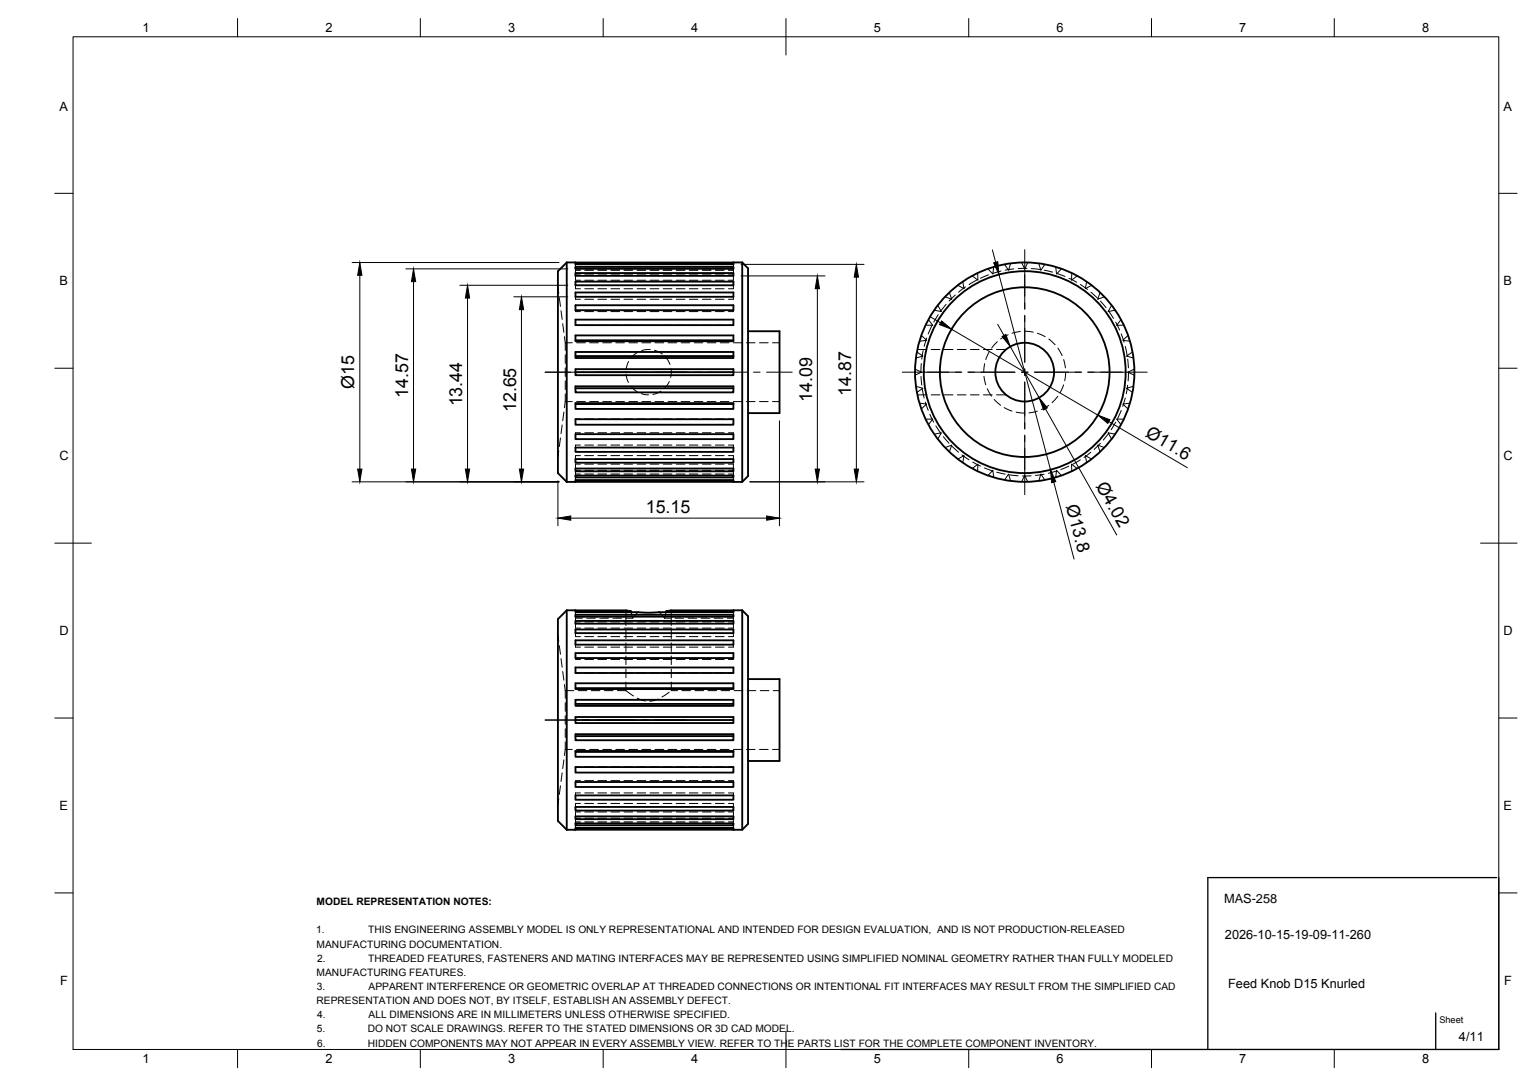
ISO-10303-21;
HEADER;
/* Generated by software containing ST-Developer
 * from STEP Tools, Inc. (www.steptools.com) 
 */

FILE_DESCRIPTION(
/* description */ (''),
/* implementation_level */ '2;1');

FILE_NAME(
/* name */ 'Feed Knob D15 Knurled.step',
/* time_stamp */ '2026-10-15T12:29:06-07:00',
/* author */ (''),
/* organization */ (''),
/* preprocessor_version */ 'ST-DEVELOPER v20.2',
/* originating_system */ 'Autodesk Translation Framework v15.15.0.0',
/* authorisation */ '');

FILE_SCHEMA (('AUTOMOTIVE_DESIGN { 1 0 10303 214 3 1 1 }'));
ENDSEC;

DATA;
#10=MECHANICAL_DESIGN_GEOMETRIC_PRESENTATION_REPRESENTATION('',(#1743),#135282);
#288=ELLIPSE('',#32479,2.77064105207217,1.55);
#289=ELLIPSE('',#32480,5.61755465834429,1.55);
#290=ELLIPSE('',#32481,3.66529504339038,1.55);
#291=ELLIPSE('',#32482,3.66529504339038,1.55);
#292=ELLIPSE('',#32483,5.6175546583443,1.55);
#293=ELLIPSE('',#32484,2.77064105207217,1.55);
#294=ELLIPSE('',#32485,2.77064105207217,1.55);
#295=ELLIPSE('',#32486,5.6175546583443,1.55);
#296=ELLIPSE('',#32487,3.66529504339038,1.55);
#297=ELLIPSE('',#32488,3.66529504339038,1.55);
#298=ELLIPSE('',#32489,5.61755465834429,1.55);
#299=ELLIPSE('',#32490,2.77064105207217,1.55);
#811=B_SPLINE_CURVE_WITH_KNOTS('',3,(#69014,#69015,#69016,#69017,#69018,
#69019),.UNSPECIFIED.,.F.,.F.,(4,2,4),(0.398092128061379,0.409976953644022,
0.468547233706402),.UNSPECIFIED.);
#812=B_SPLINE_CURVE_WITH_KNOTS('',3,(#69025,#69026,#69027,#69028,#69029,
#69030),.UNSPECIFIED.,.F.,.F.,(4,2,4),(0.254795220936954,0.292840145217421,
0.33426586804347),.UNSPECIFIED.);
#813=B_SPLINE_CURVE_WITH_KNOTS('',3,(#69036,#69037,#69038,#69039,#69040,
#69041),.UNSPECIFIED.,.F.,.F.,(4,2,4),(0.134281365662929,0.17570708848898,
0.213752012769447),.UNSPECIFIED.);
#814=B_SPLINE_CURVE_WITH_KNOTS('',3,(#69047,#69048,#69049,#69050,#69051,
#69052,#69053,#69054,#69055,#69056,#69057),.UNSPECIFIED.,.F.,.F.,(4,2,3,
2,4),(0.86663936176778,0.878524187350423,0.937094467412803,0.995664747475183,
1.00754957305783),.UNSPECIFIED.);
#815=B_SPLINE_CURVE_WITH_KNOTS('',3,(#69063,#69064,#69065,#69066,#69067,
#69068),.UNSPECIFIED.,.F.,.F.,(4,2,4),(0.723342454643356,0.761387378923823,
0.802813101749872),.UNSPECIFIED.);
#816=B_SPLINE_CURVE_WITH_KNOTS('',3,(#69074,#69075,#69076,#69077,#69078,
#69079),.UNSPECIFIED.,.F.,.F.,(4,2,4),(0.602828599369333,0.644254322195382,
0.682299246475849),.UNSPECIFIED.);
#817=B_SPLINE_CURVE_WITH_KNOTS('',3,(#69084,#69085,#69086,#69087,#69088,
#69089),.UNSPECIFIED.,.F.,.F.,(4,2,4),(0.468547233706402,0.527117513768781,
0.539002339351426),.UNSPECIFIED.);
#818=B_SPLINE_CURVE_WITH_KNOTS('',3,(#69093,#69094,#69095,#69096,#69097,
#69098,#69099,#69100,#69101,#69102,#69103,#69104,#69105,#69106,#69107,#69108,
#69109,#69110,#69111,#69112,#69113,#69114),.UNSPECIFIED.,.F.,.F.,(4,2,2,
2,2,2,2,2,2,2,4),(-0.993641732162441,-0.962200652631669,-0.930759573100898,
-0.867877414039355,-0.806554356580593,-0.745231299121831,-0.683908241663068,
-0.622585184204306,-0.559703025142763,-0.528261945611992,-0.49682086608122),
 .UNSPECIFIED.);
#819=B_SPLINE_CURVE_WITH_KNOTS('',3,(#69115,#69116,#69117,#69118,#69119,
#69120,#69121,#69122,#69123,#69124,#69125,#69126,#69127,#69128,#69129,#69130,
#69131,#69132,#69133,#69134,#69135,#69136),.UNSPECIFIED.,.F.,.F.,(4,2,2,
2,2,2,2,2,2,2,4),(-0.49682086608122,-0.465379786550449,-0.433938707019678,
-0.371056547958135,-0.309733490499373,-0.24841043304061,-0.187087375581848,
-0.125764318123086,-0.0628821590615428,-0.0314410795307714,0.),
 .UNSPECIFIED.);
#1717=SHAPE_REPRESENTATION_RELATIONSHIP('SRR','None',#135341,#1730);
#1730=ADVANCED_BREP_SHAPE_REPRESENTATION('',(#1756),#135273);
#1743=STYLED_ITEM('',(#135415),#1756);
#1756=MANIFOLD_SOLID_BREP('Body1',#32079);
#1836=CYLINDRICAL_SURFACE('',#32478,1.55);
#1837=CYLINDRICAL_SURFACE('',#32746,7.5);
#1838=CYLINDRICAL_SURFACE('',#32752,2.8);
#1839=CYLINDRICAL_SURFACE('',#32756,2.01);
#2037=FACE_BOUND('',#5476,.T.);
#2038=FACE_BOUND('',#5479,.T.);
#2039=FACE_BOUND('',#5480,.T.);
#2040=FACE_BOUND('',#5481,.T.);
#2041=FACE_BOUND('',#5482,.T.);
#2042=FACE_BOUND('',#5483,.T.);
#2043=FACE_BOUND('',#5484,.T.);
#2044=FACE_BOUND('',#5485,.T.);
#2045=FACE_BOUND('',#5486,.T.);
#2046=FACE_BOUND('',#5487,.T.);
#2047=FACE_BOUND('',#5488,.T.);
#2048=FACE_BOUND('',#5489,.T.);
#2049=FACE_BOUND('',#5490,.T.);
#2050=FACE_BOUND('',#5491,.T.);
#2051=FACE_BOUND('',#5492,.T.);
#2052=FACE_BOUND('',#5493,.T.);
#2053=FACE_BOUND('',#5494,.T.);
#2054=FACE_BOUND('',#5495,.T.);
#2055=FACE_BOUND('',#5496,.T.);
#2056=FACE_BOUND('',#5497,.T.);
#2057=FACE_BOUND('',#5498,.T.);
#2058=FACE_BOUND('',#5499,.T.);
#2059=FACE_BOUND('',#5500,.T.);
#2060=FACE_BOUND('',#5501,.T.);
#2061=FACE_BOUND('',#5502,.T.);
#2062=FACE_BOUND('',#5503,.T.);
#2063=FACE_BOUND('',#5504,.T.);
#2064=FACE_BOUND('',#5505,.T.);
#2065=FACE_BOUND('',#5506,.T.);
#2066=FACE_BOUND('',#5507,.T.);
#2067=FACE_BOUND('',#5508,.T.);
#2068=FACE_BOUND('',#5509,.T.);
#2069=FACE_BOUND('',#5510,.T.);
#2070=FACE_BOUND('',#5511,.T.);
#2071=FACE_BOUND('',#5512,.T.);
#2072=FACE_BOUND('',#5513,.T.);
#2073=FACE_BOUND('',#5514,.T.);
#2074=FACE_BOUND('',#5515,.T.);
#2075=FACE_BOUND('',#5518,.T.);
#2076=FACE_BOUND('',#5521,.T.);
#2077=FACE_BOUND('',#5523,.T.);
#2281=PLANE('',#32491);
#2282=PLANE('',#32492);
#2283=PLANE('',#32493);
#2284=PLANE('',#32494);
#2285=PLANE('',#32495);
#2286=PLANE('',#32496);
#2287=PLANE('',#32497);
#2288=PLANE('',#32498);
#2289=PLANE('',#32499);
#2290=PLANE('',#32500);
#2291=PLANE('',#32501);
#2292=PLANE('',#32503);
#2293=PLANE('',#32505);
#2294=PLANE('',#32506);
#2295=PLANE('',#32508);
#2296=PLANE('',#32509);
#2297=PLANE('',#32511);
#2298=PLANE('',#32512);
#2299=PLANE('',#32514);
#2300=PLANE('',#32515);
#2301=PLANE('',#32517);
#2302=PLANE('',#32518);
#2303=PLANE('',#32520);
#2304=PLANE('',#32521);
#2305=PLANE('',#32523);
#2306=PLANE('',#32524);
#2307=PLANE('',#32526);
#2308=PLANE('',#32527);
#2309=PLANE('',#32529);
#2310=PLANE('',#32530);
#2311=PLANE('',#32532);
#2312=PLANE('',#32533);
#2313=PLANE('',#32535);
#2314=PLANE('',#32536);
#2315=PLANE('',#32538);
#2316=PLANE('',#32539);
#2317=PLANE('',#32541);
#2318=PLANE('',#32542);
#2319=PLANE('',#32544);
#2320=PLANE('',#32545);
#2321=PLANE('',#32547);
#2322=PLANE('',#32548);
#2323=PLANE('',#32550);
#2324=PLANE('',#32551);
#2325=PLANE('',#32553);
#2326=PLANE('',#32554);
#2327=PLANE('',#32556);
#2328=PLANE('',#32557);
#2329=PLANE('',#32559);
#2330=PLANE('',#32560);
#2331=PLANE('',#32562);
#2332=PLANE('',#32563);
#2333=PLANE('',#32565);
#2334=PLANE('',#32566);
#2335=PLANE('',#32568);
#2336=PLANE('',#32569);
#2337=PLANE('',#32571);
#2338=PLANE('',#32572);
#2339=PLANE('',#32574);
#2340=PLANE('',#32575);
#2341=PLANE('',#32577);
#2342=PLANE('',#32578);
#2343=PLANE('',#32580);
#2344=PLANE('',#32581);
#2345=PLANE('',#32583);
#2346=PLANE('',#32584);
#2347=PLANE('',#32586);
#2348=PLANE('',#32587);
#2349=PLANE('',#32589);
#2350=PLANE('',#32590);
#2351=PLANE('',#32592);
#2352=PLANE('',#32593);
#2353=PLANE('',#32595);
#2354=PLANE('',#32596);
#2355=PLANE('',#32598);
#2356=PLANE('',#32599);
#2357=PLANE('',#32601);
#2358=PLANE('',#32602);
#2359=PLANE('',#32604);
#2360=PLANE('',#32605);
#2361=PLANE('',#32607);
#2362=PLANE('',#32608);
#2363=PLANE('',#32610);
#2364=PLANE('',#32611);
#2365=PLANE('',#32613);
#2366=PLANE('',#32614);
#2367=PLANE('',#32617);
#2368=PLANE('',#32618);
#2369=PLANE('',#32621);
#2370=PLANE('',#32622);
#2371=PLANE('',#32624);
#2372=PLANE('',#32625);
#2373=PLANE('',#32627);
#2374=PLANE('',#32628);
#2375=PLANE('',#32630);
#2376=PLANE('',#32631);
#2377=PLANE('',#32633);
#2378=PLANE('',#32634);
#2379=PLANE('',#32636);
#2380=PLANE('',#32637);
#2381=PLANE('',#32639);
#2382=PLANE('',#32640);
#2383=PLANE('',#32642);
#2384=PLANE('',#32643);
#2385=PLANE('',#32645);
#2386=PLANE('',#32646);
#2387=PLANE('',#32648);
#2388=PLANE('',#32649);
#2389=PLANE('',#32651);
#2390=PLANE('',#32652);
#2391=PLANE('',#32654);
#2392=PLANE('',#32655);
#2393=PLANE('',#32657);
#2394=PLANE('',#32658);
#2395=PLANE('',#32660);
#2396=PLANE('',#32661);
#2397=PLANE('',#32663);
#2398=PLANE('',#32664);
#2399=PLANE('',#32666);
#2400=PLANE('',#32667);
#2401=PLANE('',#32669);
#2402=PLANE('',#32670);
#2403=PLANE('',#32672);
#2404=PLANE('',#32673);
#2405=PLANE('',#32675);
#2406=PLANE('',#32676);
#2407=PLANE('',#32678);
#2408=PLANE('',#32679);
#2409=PLANE('',#32681);
#2410=PLANE('',#32682);
#2411=PLANE('',#32684);
#2412=PLANE('',#32685);
#2413=PLANE('',#32687);
#2414=PLANE('',#32688);
#2415=PLANE('',#32690);
#2416=PLANE('',#32691);
#2417=PLANE('',#32693);
#2418=PLANE('',#32694);
#2419=PLANE('',#32696);
#2420=PLANE('',#32697);
#2421=PLANE('',#32699);
#2422=PLANE('',#32700);
#2423=PLANE('',#32702);
#2424=PLANE('',#32703);
#2425=PLANE('',#32705);
#2426=PLANE('',#32706);
#2427=PLANE('',#32708);
#2428=PLANE('',#32709);
#2429=PLANE('',#32711);
#2430=PLANE('',#32712);
#2431=PLANE('',#32714);
#2432=PLANE('',#32715);
#2433=PLANE('',#32717);
#2434=PLANE('',#32718);
#2435=PLANE('',#32720);
#2436=PLANE('',#32721);
#2437=PLANE('',#32723);
#2438=PLANE('',#32724);
#2439=PLANE('',#32726);
#2440=PLANE('',#32727);
#2441=PLANE('',#32729);
#2442=PLANE('',#32730);
#2443=PLANE('',#32732);
#2444=PLANE('',#32733);
#2445=PLANE('',#32735);
#2446=PLANE('',#32737);
#2447=PLANE('',#32742);
#2448=PLANE('',#32750);
#2449=PLANE('',#32754);
#3532=FACE_OUTER_BOUND('',#5307,.T.);
#3533=FACE_OUTER_BOUND('',#5308,.T.);
#3534=FACE_OUTER_BOUND('',#5309,.T.);
#3535=FACE_OUTER_BOUND('',#5310,.T.);
#3536=FACE_OUTER_BOUND('',#5311,.T.);
#3537=FACE_OUTER_BOUND('',#5312,.T.);
#3538=FACE_OUTER_BOUND('',#5313,.T.);
#3539=FACE_OUTER_BOUND('',#5314,.T.);
#3540=FACE_OUTER_BOUND('',#5315,.T.);
#3541=FACE_OUTER_BOUND('',#5316,.T.);
#3542=FACE_OUTER_BOUND('',#5317,.T.);
#3543=FACE_OUTER_BOUND('',#5318,.T.);
#3544=FACE_OUTER_BOUND('',#5319,.T.);
#3545=FACE_OUTER_BOUND('',#5320,.T.);
#3546=FACE_OUTER_BOUND('',#5321,.T.);
#3547=FACE_OUTER_BOUND('',#5322,.T.);
#3548=FACE_OUTER_BOUND('',#5323,.T.);
#3549=FACE_OUTER_BOUND('',#5324,.T.);
#3550=FACE_OUTER_BOUND('',#5325,.T.);
#3551=FACE_OUTER_BOUND('',#5326,.T.);
#3552=FACE_OUTER_BOUND('',#5327,.T.);
#3553=FACE_OUTER_BOUND('',#5328,.T.);
#3554=FACE_OUTER_BOUND('',#5329,.T.);
#3555=FACE_OUTER_BOUND('',#5330,.T.);
#3556=FACE_OUTER_BOUND('',#5331,.T.);
#3557=FACE_OUTER_BOUND('',#5332,.T.);
#3558=FACE_OUTER_BOUND('',#5333,.T.);
#3559=FACE_OUTER_BOUND('',#5334,.T.);
#3560=FACE_OUTER_BOUND('',#5335,.T.);
#3561=FACE_OUTER_BOUND('',#5336,.T.);
#3562=FACE_OUTER_BOUND('',#5337,.T.);
#3563=FACE_OUTER_BOUND('',#5338,.T.);
#3564=FACE_OUTER_BOUND('',#5339,.T.);
#3565=FACE_OUTER_BOUND('',#5340,.T.);
#3566=FACE_OUTER_BOUND('',#5341,.T.);
#3567=FACE_OUTER_BOUND('',#5342,.T.);
#3568=FACE_OUTER_BOUND('',#5343,.T.);
#3569=FACE_OUTER_BOUND('',#5344,.T.);
#3570=FACE_OUTER_BOUND('',#5345,.T.);
#3571=FACE_OUTER_BOUND('',#5346,.T.);
#3572=FACE_OUTER_BOUND('',#5347,.T.);
#3573=FACE_OUTER_BOUND('',#5348,.T.);
#3574=FACE_OUTER_BOUND('',#5349,.T.);
#3575=FACE_OUTER_BOUND('',#5350,.T.);
#3576=FACE_OUTER_BOUND('',#5351,.T.);
#3577=FACE_OUTER_BOUND('',#5352,.T.);
#3578=FACE_OUTER_BOUND('',#5353,.T.);
#3579=FACE_OUTER_BOUND('',#5354,.T.);
#3580=FACE_OUTER_BOUND('',#5355,.T.);
#3581=FACE_OUTER_BOUND('',#5356,.T.);
#3582=FACE_OUTER_BOUND('',#5357,.T.);
#3583=FACE_OUTER_BOUND('',#5358,.T.);
#3584=FACE_OUTER_BOUND('',#5359,.T.);
#3585=FACE_OUTER_BOUND('',#5360,.T.);
#3586=FACE_OUTER_BOUND('',#5361,.T.);
#3587=FACE_OUTER_BOUND('',#5362,.T.);
#3588=FACE_OUTER_BOUND('',#5363,.T.);
#3589=FACE_OUTER_BOUND('',#5364,.T.);
#3590=FACE_OUTER_BOUND('',#5365,.T.);
#3591=FACE_OUTER_BOUND('',#5366,.T.);
#3592=FACE_OUTER_BOUND('',#5367,.T.);
#3593=FACE_OUTER_BOUND('',#5368,.T.);
#3594=FACE_OUTER_BOUND('',#5369,.T.);
#3595=FACE_OUTER_BOUND('',#5370,.T.);
#3596=FACE_OUTER_BOUND('',#5371,.T.);
#3597=FACE_OUTER_BOUND('',#5372,.T.);
#3598=FACE_OUTER_BOUND('',#5373,.T.);
#3599=FACE_OUTER_BOUND('',#5374,.T.);
#3600=FACE_OUTER_BOUND('',#5375,.T.);
#3601=FACE_OUTER_BOUND('',#5376,.T.);
#3602=FACE_OUTER_BOUND('',#5377,.T.);
#3603=FACE_OUTER_BOUND('',#5378,.T.);
#3604=FACE_OUTER_BOUND('',#5379,.T.);
#3605=FACE_OUTER_BOUND('',#5380,.T.);
#3606=FACE_OUTER_BOUND('',#5381,.T.);
#3607=FACE_OUTER_BOUND('',#5382,.T.);
#3608=FACE_OUTER_BOUND('',#5383,.T.);
#3609=FACE_OUTER_BOUND('',#5384,.T.);
#3610=FACE_OUTER_BOUND('',#5385,.T.);
#3611=FACE_OUTER_BOUND('',#5386,.T.);
#3612=FACE_OUTER_BOUND('',#5387,.T.);
#3613=FACE_OUTER_BOUND('',#5388,.T.);
#3614=FACE_OUTER_BOUND('',#5389,.T.);
#3615=FACE_OUTER_BOUND('',#5390,.T.);
#3616=FACE_OUTER_BOUND('',#5391,.T.);
#3617=FACE_OUTER_BOUND('',#5392,.T.);
#3618=FACE_OUTER_BOUND('',#5393,.T.);
#3619=FACE_OUTER_BOUND('',#5394,.T.);
#3620=FACE_OUTER_BOUND('',#5395,.T.);
#3621=FACE_OUTER_BOUND('',#5396,.T.);
#3622=FACE_OUTER_BOUND('',#5397,.T.);
#3623=FACE_OUTER_BOUND('',#5398,.T.);
#3624=FACE_OUTER_BOUND('',#5399,.T.);
#3625=FACE_OUTER_BOUND('',#5400,.T.);
#3626=FACE_OUTER_BOUND('',#5401,.T.);
#3627=FACE_OUTER_BOUND('',#5402,.T.);
#3628=FACE_OUTER_BOUND('',#5403,.T.);
#3629=FACE_OUTER_BOUND('',#5404,.T.);
#3630=FACE_OUTER_BOUND('',#5405,.T.);
#3631=FACE_OUTER_BOUND('',#5406,.T.);
#3632=FACE_OUTER_BOUND('',#5407,.T.);
#3633=FACE_OUTER_BOUND('',#5408,.T.);
#3634=FACE_OUTER_BOUND('',#5409,.T.);
#3635=FACE_OUTER_BOUND('',#5410,.T.);
#3636=FACE_OUTER_BOUND('',#5411,.T.);
#3637=FACE_OUTER_BOUND('',#5412,.T.);
#3638=FACE_OUTER_BOUND('',#5413,.T.);
#3639=FACE_OUTER_BOUND('',#5414,.T.);
#3640=FACE_OUTER_BOUND('',#5415,.T.);
#3641=FACE_OUTER_BOUND('',#5416,.T.);
#3642=FACE_OUTER_BOUND('',#5417,.T.);
#3643=FACE_OUTER_BOUND('',#5418,.T.);
#3644=FACE_OUTER_BOUND('',#5419,.T.);
#3645=FACE_OUTER_BOUND('',#5420,.T.);
#3646=FACE_OUTER_BOUND('',#5421,.T.);
#3647=FACE_OUTER_BOUND('',#5422,.T.);
#3648=FACE_OUTER_BOUND('',#5423,.T.);
#3649=FACE_OUTER_BOUND('',#5424,.T.);
#3650=FACE_OUTER_BOUND('',#5425,.T.);
#3651=FACE_OUTER_BOUND('',#5426,.T.);
#3652=FACE_OUTER_BOUND('',#5427,.T.);
#3653=FACE_OUTER_BOUND('',#5428,.T.);
#3654=FACE_OUTER_BOUND('',#5429,.T.);
#3655=FACE_OUTER_BOUND('',#5430,.T.);
#3656=FACE_OUTER_BOUND('',#5431,.T.);
#3657=FACE_OUTER_BOUND('',#5432,.T.);
#3658=FACE_OUTER_BOUND('',#5433,.T.);
#3659=FACE_OUTER_BOUND('',#5434,.T.);
#3660=FACE_OUTER_BOUND('',#5435,.T.);
#3661=FACE_OUTER_BOUND('',#5436,.T.);
#3662=FACE_OUTER_BOUND('',#5437,.T.);
#3663=FACE_OUTER_BOUND('',#5438,.T.);
#3664=FACE_OUTER_BOUND('',#5439,.T.);
#3665=FACE_OUTER_BOUND('',#5440,.T.);
#3666=FACE_OUTER_BOUND('',#5441,.T.);
#3667=FACE_OUTER_BOUND('',#5442,.T.);
#3668=FACE_OUTER_BOUND('',#5443,.T.);
#3669=FACE_OUTER_BOUND('',#5444,.T.);
#3670=FACE_OUTER_BOUND('',#5445,.T.);
#3671=FACE_OUTER_BOUND('',#5446,.T.);
#3672=FACE_OUTER_BOUND('',#5447,.T.);
#3673=FACE_OUTER_BOUND('',#5448,.T.);
#3674=FACE_OUTER_BOUND('',#5449,.T.);
#3675=FACE_OUTER_BOUND('',#5450,.T.);
#3676=FACE_OUTER_BOUND('',#5451,.T.);
#3677=FACE_OUTER_BOUND('',#5452,.T.);
#3678=FACE_OUTER_BOUND('',#5453,.T.);
#3679=FACE_OUTER_BOUND('',#5454,.T.);
#3680=FACE_OUTER_BOUND('',#5455,.T.);
#3681=FACE_OUTER_BOUND('',#5456,.T.);
#3682=FACE_OUTER_BOUND('',#5457,.T.);
#3683=FACE_OUTER_BOUND('',#5458,.T.);
#3684=FACE_OUTER_BOUND('',#5459,.T.);
#3685=FACE_OUTER_BOUND('',#5460,.T.);
#3686=FACE_OUTER_BOUND('',#5461,.T.);
#3687=FACE_OUTER_BOUND('',#5462,.T.);
#3688=FACE_OUTER_BOUND('',#5463,.T.);
#3689=FACE_OUTER_BOUND('',#5464,.T.);
#3690=FACE_OUTER_BOUND('',#5465,.T.);
#3691=FACE_OUTER_BOUND('',#5466,.T.);
#3692=FACE_OUTER_BOUND('',#5467,.T.);
#3693=FACE_OUTER_BOUND('',#5468,.T.);
#3694=FACE_OUTER_BOUND('',#5469,.T.);
#3695=FACE_OUTER_BOUND('',#5470,.T.);
#3696=FACE_OUTER_BOUND('',#5471,.T.);
#3697=FACE_OUTER_BOUND('',#5472,.T.);
#3698=FACE_OUTER_BOUND('',#5473,.T.);
#3699=FACE_OUTER_BOUND('',#5474,.T.);
#3700=FACE_OUTER_BOUND('',#5475,.T.);
#3701=FACE_OUTER_BOUND('',#5477,.T.);
#3702=FACE_OUTER_BOUND('',#5478,.T.);
#3703=FACE_OUTER_BOUND('',#5516,.T.);
#3704=FACE_OUTER_BOUND('',#5517,.T.);
#3705=FACE_OUTER_BOUND('',#5519,.T.);
#3706=FACE_OUTER_BOUND('',#5520,.T.);
#3707=FACE_OUTER_BOUND('',#5522,.T.);
#5307=EDGE_LOOP('',(#21964,#21965,#21966,#21967,#21968,#21969,#21970,#21971,
#21972,#21973,#21974,#21975,#21976,#21977,#21978,#21979,#21980,#21981,#21982,
#21983,#21984,#21985,#21986));
#5308=EDGE_LOOP('',(#21987,#21988,#21989,#21990));
#5309=EDGE_LOOP('',(#21991,#21992,#21993,#21994));
#5310=EDGE_LOOP('',(#21995,#21996,#21997,#21998));
#5311=EDGE_LOOP('',(#21999,#22000,#22001,#22002));
#5312=EDGE_LOOP('',(#22003,#22004,#22005,#22006));
#5313=EDGE_LOOP('',(#22007,#22008,#22009,#22010));
#5314=EDGE_LOOP('',(#22011,#22012,#22013,#22014));
#5315=EDGE_LOOP('',(#22015,#22016,#22017,#22018));
#5316=EDGE_LOOP('',(#22019,#22020,#22021,#22022));
#5317=EDGE_LOOP('',(#22023,#22024,#22025,#22026));
#5318=EDGE_LOOP('',(#22027,#22028,#22029));
#5319=EDGE_LOOP('',(#22030,#22031,#22032));
#5320=EDGE_LOOP('',(#22033,#22034,#22035,#22036));
#5321=EDGE_LOOP('',(#22037,#22038,#22039));
#5322=EDGE_LOOP('',(#22040,#22041,#22042,#22043));
#5323=EDGE_LOOP('',(#22044,#22045,#22046));
#5324=EDGE_LOOP('',(#22047,#22048,#22049,#22050));
#5325=EDGE_LOOP('',(#22051,#22052,#22053));
#5326=EDGE_LOOP('',(#22054,#22055,#22056,#22057));
#5327=EDGE_LOOP('',(#22058,#22059,#22060));
#5328=EDGE_LOOP('',(#22061,#22062,#22063,#22064));
#5329=EDGE_LOOP('',(#22065,#22066,#22067));
#5330=EDGE_LOOP('',(#22068,#22069,#22070,#22071));
#5331=EDGE_LOOP('',(#22072,#22073,#22074));
#5332=EDGE_LOOP('',(#22075,#22076,#22077,#22078));
#5333=EDGE_LOOP('',(#22079,#22080,#22081));
#5334=EDGE_LOOP('',(#22082,#22083,#22084,#22085));
#5335=EDGE_LOOP('',(#22086,#22087,#22088));
#5336=EDGE_LOOP('',(#22089,#22090,#22091,#22092));
#5337=EDGE_LOOP('',(#22093,#22094,#22095));
#5338=EDGE_LOOP('',(#22096,#22097,#22098,#22099));
#5339=EDGE_LOOP('',(#22100,#22101,#22102));
#5340=EDGE_LOOP('',(#22103,#22104,#22105,#22106));
#5341=EDGE_LOOP('',(#22107,#22108,#22109));
#5342=EDGE_LOOP('',(#22110,#22111,#22112,#22113));
#5343=EDGE_LOOP('',(#22114,#22115,#22116));
#5344=EDGE_LOOP('',(#22117,#22118,#22119,#22120));
#5345=EDGE_LOOP('',(#22121,#22122,#22123));
#5346=EDGE_LOOP('',(#22124,#22125,#22126,#22127));
#5347=EDGE_LOOP('',(#22128,#22129,#22130));
#5348=EDGE_LOOP('',(#22131,#22132,#22133,#22134));
#5349=EDGE_LOOP('',(#22135,#22136,#22137));
#5350=EDGE_LOOP('',(#22138,#22139,#22140,#22141));
#5351=EDGE_LOOP('',(#22142,#22143,#22144));
#5352=EDGE_LOOP('',(#22145,#22146,#22147,#22148));
#5353=EDGE_LOOP('',(#22149,#22150,#22151));
#5354=EDGE_LOOP('',(#22152,#22153,#22154,#22155));
#5355=EDGE_LOOP('',(#22156,#22157,#22158));
#5356=EDGE_LOOP('',(#22159,#22160,#22161,#22162));
#5357=EDGE_LOOP('',(#22163,#22164,#22165));
#5358=EDGE_LOOP('',(#22166,#22167,#22168,#22169));
#5359=EDGE_LOOP('',(#22170,#22171,#22172));
#5360=EDGE_LOOP('',(#22173,#22174,#22175,#22176));
#5361=EDGE_LOOP('',(#22177,#22178,#22179));
#5362=EDGE_LOOP('',(#22180,#22181,#22182,#22183));
#5363=EDGE_LOOP('',(#22184,#22185,#22186));
#5364=EDGE_LOOP('',(#22187,#22188,#22189,#22190));
#5365=EDGE_LOOP('',(#22191,#22192,#22193));
#5366=EDGE_LOOP('',(#22194,#22195,#22196,#22197));
#5367=EDGE_LOOP('',(#22198,#22199,#22200));
#5368=EDGE_LOOP('',(#22201,#22202,#22203,#22204));
#5369=EDGE_LOOP('',(#22205,#22206,#22207));
#5370=EDGE_LOOP('',(#22208,#22209,#22210,#22211));
#5371=EDGE_LOOP('',(#22212,#22213,#22214));
#5372=EDGE_LOOP('',(#22215,#22216,#22217,#22218));
#5373=EDGE_LOOP('',(#22219,#22220,#22221));
#5374=EDGE_LOOP('',(#22222,#22223,#22224,#22225));
#5375=EDGE_LOOP('',(#22226,#22227,#22228));
#5376=EDGE_LOOP('',(#22229,#22230,#22231,#22232));
#5377=EDGE_LOOP('',(#22233,#22234,#22235));
#5378=EDGE_LOOP('',(#22236,#22237,#22238,#22239));
#5379=EDGE_LOOP('',(#22240,#22241,#22242));
#5380=EDGE_LOOP('',(#22243,#22244,#22245,#22246));
#5381=EDGE_LOOP('',(#22247,#22248,#22249));
#5382=EDGE_LOOP('',(#22250,#22251,#22252,#22253));
#5383=EDGE_LOOP('',(#22254,#22255,#22256));
#5384=EDGE_LOOP('',(#22257,#22258,#22259,#22260));
#5385=EDGE_LOOP('',(#22261,#22262,#22263));
#5386=EDGE_LOOP('',(#22264,#22265,#22266,#22267));
#5387=EDGE_LOOP('',(#22268,#22269,#22270));
#5388=EDGE_LOOP('',(#22271,#22272,#22273,#22274));
#5389=EDGE_LOOP('',(#22275,#22276,#22277));
#5390=EDGE_LOOP('',(#22278,#22279,#22280,#22281));
#5391=EDGE_LOOP('',(#22282,#22283,#22284));
#5392=EDGE_LOOP('',(#22285,#22286,#22287,#22288));
#5393=EDGE_LOOP('',(#22289,#22290,#22291,#22292));
#5394=EDGE_LOOP('',(#22293,#22294,#22295,#22296));
#5395=EDGE_LOOP('',(#22297,#22298,#22299,#22300));
#5396=EDGE_LOOP('',(#22301,#22302,#22303,#22304));
#5397=EDGE_LOOP('',(#22305,#22306,#22307));
#5398=EDGE_LOOP('',(#22308,#22309,#22310,#22311));
#5399=EDGE_LOOP('',(#22312,#22313,#22314));
#5400=EDGE_LOOP('',(#22315,#22316,#22317,#22318));
#5401=EDGE_LOOP('',(#22319,#22320,#22321));
#5402=EDGE_LOOP('',(#22322,#22323,#22324,#22325));
#5403=EDGE_LOOP('',(#22326,#22327,#22328));
#5404=EDGE_LOOP('',(#22329,#22330,#22331,#22332));
#5405=EDGE_LOOP('',(#22333,#22334,#22335));
#5406=EDGE_LOOP('',(#22336,#22337,#22338,#22339));
#5407=EDGE_LOOP('',(#22340,#22341,#22342));
#5408=EDGE_LOOP('',(#22343,#22344,#22345,#22346));
#5409=EDGE_LOOP('',(#22347,#22348,#22349));
#5410=EDGE_LOOP('',(#22350,#22351,#22352,#22353));
#5411=EDGE_LOOP('',(#22354,#22355,#22356));
#5412=EDGE_LOOP('',(#22357,#22358,#22359,#22360));
#5413=EDGE_LOOP('',(#22361,#22362,#22363));
#5414=EDGE_LOOP('',(#22364,#22365,#22366,#22367));
#5415=EDGE_LOOP('',(#22368,#22369,#22370));
#5416=EDGE_LOOP('',(#22371,#22372,#22373,#22374));
#5417=EDGE_LOOP('',(#22375,#22376,#22377));
#5418=EDGE_LOOP('',(#22378,#22379,#22380,#22381));
#5419=EDGE_LOOP('',(#22382,#22383,#22384));
#5420=EDGE_LOOP('',(#22385,#22386,#22387,#22388));
#5421=EDGE_LOOP('',(#22389,#22390,#22391));
#5422=EDGE_LOOP('',(#22392,#22393,#22394,#22395));
#5423=EDGE_LOOP('',(#22396,#22397,#22398));
#5424=EDGE_LOOP('',(#22399,#22400,#22401,#22402));
#5425=EDGE_LOOP('',(#22403,#22404,#22405));
#5426=EDGE_LOOP('',(#22406,#22407,#22408,#22409));
#5427=EDGE_LOOP('',(#22410,#22411,#22412));
#5428=EDGE_LOOP('',(#22413,#22414,#22415,#22416));
#5429=EDGE_LOOP('',(#22417,#22418,#22419));
#5430=EDGE_LOOP('',(#22420,#22421,#22422,#22423));
#5431=EDGE_LOOP('',(#22424,#22425,#22426));
#5432=EDGE_LOOP('',(#22427,#22428,#22429,#22430));
#5433=EDGE_LOOP('',(#22431,#22432,#22433));
#5434=EDGE_LOOP('',(#22434,#22435,#22436,#22437));
#5435=EDGE_LOOP('',(#22438,#22439,#22440));
#5436=EDGE_LOOP('',(#22441,#22442,#22443,#22444));
#5437=EDGE_LOOP('',(#22445,#22446,#22447));
#5438=EDGE_LOOP('',(#22448,#22449,#22450,#22451));
#5439=EDGE_LOOP('',(#22452,#22453,#22454));
#5440=EDGE_LOOP('',(#22455,#22456,#22457,#22458));
#5441=EDGE_LOOP('',(#22459,#22460,#22461));
#5442=EDGE_LOOP('',(#22462,#22463,#22464,#22465));
#5443=EDGE_LOOP('',(#22466,#22467,#22468));
#5444=EDGE_LOOP('',(#22469,#22470,#22471,#22472));
#5445=EDGE_LOOP('',(#22473,#22474,#22475));
#5446=EDGE_LOOP('',(#22476,#22477,#22478,#22479));
#5447=EDGE_LOOP('',(#22480,#22481,#22482));
#5448=EDGE_LOOP('',(#22483,#22484,#22485,#22486));
#5449=EDGE_LOOP('',(#22487,#22488,#22489));
#5450=EDGE_LOOP('',(#22490,#22491,#22492,#22493));
#5451=EDGE_LOOP('',(#22494,#22495,#22496));
#5452=EDGE_LOOP('',(#22497,#22498,#22499,#22500));
#5453=EDGE_LOOP('',(#22501,#22502,#22503));
#5454=EDGE_LOOP('',(#22504,#22505,#22506,#22507));
#5455=EDGE_LOOP('',(#22508,#22509,#22510));
#5456=EDGE_LOOP('',(#22511,#22512,#22513,#22514));
#5457=EDGE_LOOP('',(#22515,#22516,#22517));
#5458=EDGE_LOOP('',(#22518,#22519,#22520,#22521));
#5459=EDGE_LOOP('',(#22522,#22523,#22524));
#5460=EDGE_LOOP('',(#22525,#22526,#22527,#22528));
#5461=EDGE_LOOP('',(#22529,#22530,#22531));
#5462=EDGE_LOOP('',(#22532,#22533,#22534,#22535));
#5463=EDGE_LOOP('',(#22536,#22537,#22538));
#5464=EDGE_LOOP('',(#22539,#22540,#22541,#22542));
#5465=EDGE_LOOP('',(#22543,#22544,#22545));
#5466=EDGE_LOOP('',(#22546,#22547,#22548,#22549));
#5467=EDGE_LOOP('',(#22550,#22551,#22552));
#5468=EDGE_LOOP('',(#22553,#22554,#22555,#22556));
#5469=EDGE_LOOP('',(#22557,#22558,#22559));
#5470=EDGE_LOOP('',(#22560,#22561,#22562,#22563));
#5471=EDGE_LOOP('',(#22564,#22565,#22566));
#5472=EDGE_LOOP('',(#22567,#22568,#22569));
#5473=EDGE_LOOP('',(#22570,#22571,#22572));
#5474=EDGE_LOOP('',(#22573,#22574,#22575,#22576));
#5475=EDGE_LOOP('',(#22577));
#5476=EDGE_LOOP('',(#22578));
#5477=EDGE_LOOP('',(#22579,#22580,#22581,#22582));
#5478=EDGE_LOOP('',(#22583,#22584,#22585,#22586,#22587,#22588,#22589,#22590,
#22591,#22592,#22593,#22594));
#5479=EDGE_LOOP('',(#22595,#22596,#22597,#22598,#22599,#22600,#22601,#22602,
#22603,#22604,#22605,#22606,#22607,#22608,#22609,#22610,#22611,#22612,#22613,
#22614,#22615,#22616,#22617,#22618,#22619));
#5480=EDGE_LOOP('',(#22620,#22621,#22622,#22623));
#5481=EDGE_LOOP('',(#22624,#22625,#22626,#22627));
#5482=EDGE_LOOP('',(#22628,#22629,#22630,#22631));
#5483=EDGE_LOOP('',(#22632,#22633,#22634,#22635));
#5484=EDGE_LOOP('',(#22636,#22637,#22638,#22639));
#5485=EDGE_LOOP('',(#22640,#22641,#22642,#22643));
#5486=EDGE_LOOP('',(#22644,#22645,#22646,#22647));
#5487=EDGE_LOOP('',(#22648,#22649,#22650,#22651));
#5488=EDGE_LOOP('',(#22652,#22653,#22654,#22655));
#5489=EDGE_LOOP('',(#22656,#22657,#22658,#22659));
#5490=EDGE_LOOP('',(#22660,#22661,#22662,#22663));
#5491=EDGE_LOOP('',(#22664,#22665,#22666,#22667));
#5492=EDGE_LOOP('',(#22668,#22669,#22670,#22671));
#5493=EDGE_LOOP('',(#22672,#22673,#22674,#22675));
#5494=EDGE_LOOP('',(#22676,#22677,#22678,#22679));
#5495=EDGE_LOOP('',(#22680,#22681,#22682,#22683));
#5496=EDGE_LOOP('',(#22684,#22685,#22686,#22687));
#5497=EDGE_LOOP('',(#22688,#22689,#22690,#22691));
#5498=EDGE_LOOP('',(#22692,#22693,#22694,#22695));
#5499=EDGE_LOOP('',(#22696,#22697,#22698,#22699));
#5500=EDGE_LOOP('',(#22700,#22701,#22702,#22703));
#5501=EDGE_LOOP('',(#22704,#22705,#22706,#22707));
#5502=EDGE_LOOP('',(#22708,#22709,#22710,#22711));
#5503=EDGE_LOOP('',(#22712,#22713,#22714,#22715));
#5504=EDGE_LOOP('',(#22716,#22717,#22718,#22719));
#5505=EDGE_LOOP('',(#22720,#22721,#22722,#22723));
#5506=EDGE_LOOP('',(#22724,#22725,#22726,#22727));
#5507=EDGE_LOOP('',(#22728,#22729,#22730,#22731));
#5508=EDGE_LOOP('',(#22732,#22733,#22734,#22735));
#5509=EDGE_LOOP('',(#22736,#22737,#22738,#22739));
#5510=EDGE_LOOP('',(#22740,#22741,#22742,#22743));
#5511=EDGE_LOOP('',(#22744,#22745,#22746,#22747));
#5512=EDGE_LOOP('',(#22748,#22749,#22750,#22751));
#5513=EDGE_LOOP('',(#22752,#22753,#22754,#22755));
#5514=EDGE_LOOP('',(#22756,#22757,#22758,#22759));
#5515=EDGE_LOOP('',(#22760,#22761,#22762,#22763));
#5516=EDGE_LOOP('',(#22764,#22765,#22766,#22767));
#5517=EDGE_LOOP('',(#22768));
#5518=EDGE_LOOP('',(#22769));
#5519=EDGE_LOOP('',(#22770,#22771,#22772,#22773));
#5520=EDGE_LOOP('',(#22774));
#5521=EDGE_LOOP('',(#22775));
#5522=EDGE_LOOP('',(#22776,#22777,#22778,#22779));
#5523=EDGE_LOOP('',(#22780,#22781));
#7289=LINE('',#69091,#10126);
#7290=LINE('',#69139,#10127);
#7291=LINE('',#69141,#10128);
#7292=LINE('',#69142,#10129);
#7293=LINE('',#69145,#10130);
#7294=LINE('',#69146,#10131);
#7295=LINE('',#69149,#10132);
#7296=LINE('',#69151,#10133);
#7297=LINE('',#69152,#10134);
#7298=LINE('',#69155,#10135);
#7299=LINE('',#69157,#10136);
#7300=LINE('',#69158,#10137);
#7301=LINE('',#69161,#10138);
#7302=LINE('',#69162,#10139);
#7303=LINE('',#69165,#10140);
#7304=LINE('',#69166,#10141);
#7305=LINE('',#69169,#10142);
#7306=LINE('',#69171,#10143);
#7307=LINE('',#69172,#10144);
#7308=LINE('',#69175,#10145);
#7309=LINE('',#69177,#10146);
#7310=LINE('',#69178,#10147);
#7311=LINE('',#69181,#10148);
#7312=LINE('',#69182,#10149);
#7313=LINE('',#69185,#10150);
#7314=LINE('',#69186,#10151);
#7315=LINE('',#69194,#10152);
#7316=LINE('',#69196,#10153);
#7317=LINE('',#69198,#10154);
#7318=LINE('',#69199,#10155);
#7319=LINE('',#69203,#10156);
#7320=LINE('',#69206,#10157);
#7321=LINE('',#69207,#10158);
#7322=LINE('',#69213,#10159);
#7323=LINE('',#69215,#10160);
#7324=LINE('',#69217,#10161);
#7325=LINE('',#69218,#10162);
#7326=LINE('',#69222,#10163);
#7327=LINE('',#69225,#10164);
#7328=LINE('',#69226,#10165);
#7329=LINE('',#69232,#10166);
#7330=LINE('',#69234,#10167);
#7331=LINE('',#69236,#10168);
#7332=LINE('',#69237,#10169);
#7333=LINE('',#69241,#10170);
#7334=LINE('',#69244,#10171);
#7335=LINE('',#69245,#10172);
#7336=LINE('',#69251,#10173);
#7337=LINE('',#69253,#10174);
#7338=LINE('',#69255,#10175);
#7339=LINE('',#69256,#10176);
#7340=LINE('',#69260,#10177);
#7341=LINE('',#69263,#10178);
#7342=LINE('',#69264,#10179);
#7343=LINE('',#69270,#10180);
#7344=LINE('',#69272,#10181);
#7345=LINE('',#69274,#10182);
#7346=LINE('',#69275,#10183);
#7347=LINE('',#69279,#10184);
#7348=LINE('',#69282,#10185);
#7349=LINE('',#69283,#10186);
#7350=LINE('',#69289,#10187);
#7351=LINE('',#69291,#10188);
#7352=LINE('',#69293,#10189);
#7353=LINE('',#69294,#10190);
#7354=LINE('',#69298,#10191);
#7355=LINE('',#69301,#10192);
#7356=LINE('',#69302,#10193);
#7357=LINE('',#69308,#10194);
#7358=LINE('',#69310,#10195);
#7359=LINE('',#69312,#10196);
#7360=LINE('',#69313,#10197);
#7361=LINE('',#69317,#10198);
#7362=LINE('',#69320,#10199);
#7363=LINE('',#69321,#10200);
#7364=LINE('',#69327,#10201);
#7365=LINE('',#69329,#10202);
#7366=LINE('',#69331,#10203);
#7367=LINE('',#69332,#10204);
#7368=LINE('',#69336,#10205);
#7369=LINE('',#69339,#10206);
#7370=LINE('',#69340,#10207);
#7371=LINE('',#69346,#10208);
#7372=LINE('',#69348,#10209);
#7373=LINE('',#69350,#10210);
#7374=LINE('',#69351,#10211);
#7375=LINE('',#69355,#10212);
#7376=LINE('',#69358,#10213);
#7377=LINE('',#69359,#10214);
#7378=LINE('',#69365,#10215);
#7379=LINE('',#69367,#10216);
#7380=LINE('',#69369,#10217);
#7381=LINE('',#69370,#10218);
#7382=LINE('',#69374,#10219);
#7383=LINE('',#69377,#10220);
#7384=LINE('',#69378,#10221);
#7385=LINE('',#69384,#10222);
#7386=LINE('',#69386,#10223);
#7387=LINE('',#69388,#10224);
#7388=LINE('',#69389,#10225);
#7389=LINE('',#69393,#10226);
#7390=LINE('',#69396,#10227);
#7391=LINE('',#69397,#10228);
#7392=LINE('',#69403,#10229);
#7393=LINE('',#69405,#10230);
#7394=LINE('',#69407,#10231);
#7395=LINE('',#69408,#10232);
#7396=LINE('',#69412,#10233);
#7397=LINE('',#69415,#10234);
#7398=LINE('',#69416,#10235);
#7399=LINE('',#69422,#10236);
#7400=LINE('',#69424,#10237);
#7401=LINE('',#69426,#10238);
#7402=LINE('',#69427,#10239);
#7403=LINE('',#69431,#10240);
#7404=LINE('',#69434,#10241);
#7405=LINE('',#69435,#10242);
#7406=LINE('',#69441,#10243);
#7407=LINE('',#69443,#10244);
#7408=LINE('',#69445,#10245);
#7409=LINE('',#69446,#10246);
#7410=LINE('',#69450,#10247);
#7411=LINE('',#69453,#10248);
#7412=LINE('',#69454,#10249);
#7413=LINE('',#69460,#10250);
#7414=LINE('',#69462,#10251);
#7415=LINE('',#69464,#10252);
#7416=LINE('',#69465,#10253);
#7417=LINE('',#69469,#10254);
#7418=LINE('',#69472,#10255);
#7419=LINE('',#69473,#10256);
#7420=LINE('',#69479,#10257);
#7421=LINE('',#69481,#10258);
#7422=LINE('',#69483,#10259);
#7423=LINE('',#69484,#10260);
#7424=LINE('',#69488,#10261);
#7425=LINE('',#69491,#10262);
#7426=LINE('',#69492,#10263);
#7427=LINE('',#69498,#10264);
#7428=LINE('',#69500,#10265);
#7429=LINE('',#69502,#10266);
#7430=LINE('',#69503,#10267);
#7431=LINE('',#69507,#10268);
#7432=LINE('',#69510,#10269);
#7433=LINE('',#69511,#10270);
#7434=LINE('',#69517,#10271);
#7435=LINE('',#69519,#10272);
#7436=LINE('',#69521,#10273);
#7437=LINE('',#69522,#10274);
#7438=LINE('',#69526,#10275);
#7439=LINE('',#69529,#10276);
#7440=LINE('',#69530,#10277);
#7441=LINE('',#69536,#10278);
#7442=LINE('',#69538,#10279);
#7443=LINE('',#69540,#10280);
#7444=LINE('',#69541,#10281);
#7445=LINE('',#69546,#10282);
#7446=LINE('',#69550,#10283);
#7447=LINE('',#69551,#10284);
#7448=LINE('',#69559,#10285);
#7449=LINE('',#69561,#10286);
#7450=LINE('',#69563,#10287);
#7451=LINE('',#69564,#10288);
#7452=LINE('',#69568,#10289);
#7453=LINE('',#69571,#10290);
#7454=LINE('',#69572,#10291);
#7455=LINE('',#69578,#10292);
#7456=LINE('',#69580,#10293);
#7457=LINE('',#69582,#10294);
#7458=LINE('',#69583,#10295);
#7459=LINE('',#69587,#10296);
#7460=LINE('',#69590,#10297);
#7461=LINE('',#69591,#10298);
#7462=LINE('',#69597,#10299);
#7463=LINE('',#69599,#10300);
#7464=LINE('',#69601,#10301);
#7465=LINE('',#69602,#10302);
#7466=LINE('',#69606,#10303);
#7467=LINE('',#69609,#10304);
#7468=LINE('',#69610,#10305);
#7469=LINE('',#69616,#10306);
#7470=LINE('',#69618,#10307);
#7471=LINE('',#69620,#10308);
#7472=LINE('',#69621,#10309);
#7473=LINE('',#69625,#10310);
#7474=LINE('',#69628,#10311);
#7475=LINE('',#69629,#10312);
#7476=LINE('',#69635,#10313);
#7477=LINE('',#69637,#10314);
#7478=LINE('',#69639,#10315);
#7479=LINE('',#69640,#10316);
#7480=LINE('',#69644,#10317);
#7481=LINE('',#69647,#10318);
#7482=LINE('',#69648,#10319);
#7483=LINE('',#69654,#10320);
#7484=LINE('',#69656,#10321);
#7485=LINE('',#69658,#10322);
#7486=LINE('',#69659,#10323);
#7487=LINE('',#69663,#10324);
#7488=LINE('',#69666,#10325);
#7489=LINE('',#69667,#10326);
#7490=LINE('',#69673,#10327);
#7491=LINE('',#69675,#10328);
#7492=LINE('',#69677,#10329);
#7493=LINE('',#69678,#10330);
#7494=LINE('',#69682,#10331);
#7495=LINE('',#69685,#10332);
#7496=LINE('',#69686,#10333);
#7497=LINE('',#69692,#10334);
#7498=LINE('',#69694,#10335);
#7499=LINE('',#69696,#10336);
#7500=LINE('',#69697,#10337);
#7501=LINE('',#69701,#10338);
#7502=LINE('',#69704,#10339);
#7503=LINE('',#69705,#10340);
#7504=LINE('',#69711,#10341);
#7505=LINE('',#69713,#10342);
#7506=LINE('',#69715,#10343);
#7507=LINE('',#69716,#10344);
#7508=LINE('',#69720,#10345);
#7509=LINE('',#69723,#10346);
#7510=LINE('',#69724,#10347);
#7511=LINE('',#69730,#10348);
#7512=LINE('',#69732,#10349);
#7513=LINE('',#69734,#10350);
#7514=LINE('',#69735,#10351);
#7515=LINE('',#69739,#10352);
#7516=LINE('',#69742,#10353);
#7517=LINE('',#69743,#10354);
#7518=LINE('',#69749,#10355);
#7519=LINE('',#69751,#10356);
#7520=LINE('',#69753,#10357);
#7521=LINE('',#69754,#10358);
#7522=LINE('',#69758,#10359);
#7523=LINE('',#69761,#10360);
#7524=LINE('',#69762,#10361);
#7525=LINE('',#69768,#10362);
#7526=LINE('',#69770,#10363);
#7527=LINE('',#69772,#10364);
#7528=LINE('',#69773,#10365);
#7529=LINE('',#69777,#10366);
#7530=LINE('',#69780,#10367);
#7531=LINE('',#69781,#10368);
#7532=LINE('',#69787,#10369);
#7533=LINE('',#69789,#10370);
#7534=LINE('',#69791,#10371);
#7535=LINE('',#69792,#10372);
#7536=LINE('',#69796,#10373);
#7537=LINE('',#69799,#10374);
#7538=LINE('',#69800,#10375);
#7539=LINE('',#69806,#10376);
#7540=LINE('',#69808,#10377);
#7541=LINE('',#69810,#10378);
#7542=LINE('',#69811,#10379);
#7543=LINE('',#69815,#10380);
#7544=LINE('',#69818,#10381);
#7545=LINE('',#69819,#10382);
#7546=LINE('',#69825,#10383);
#7547=LINE('',#69827,#10384);
#7548=LINE('',#69829,#10385);
#7549=LINE('',#69830,#10386);
#7550=LINE('',#69834,#10387);
#7551=LINE('',#69837,#10388);
#7552=LINE('',#69838,#10389);
#7553=LINE('',#69844,#10390);
#7554=LINE('',#69846,#10391);
#7555=LINE('',#69848,#10392);
#7556=LINE('',#69849,#10393);
#7557=LINE('',#69853,#10394);
#7558=LINE('',#69856,#10395);
#7559=LINE('',#69857,#10396);
#7560=LINE('',#69863,#10397);
#7561=LINE('',#69865,#10398);
#7562=LINE('',#69867,#10399);
#7563=LINE('',#69868,#10400);
#7564=LINE('',#69872,#10401);
#7565=LINE('',#69875,#10402);
#7566=LINE('',#69876,#10403);
#7567=LINE('',#69882,#10404);
#7568=LINE('',#69884,#10405);
#7569=LINE('',#69886,#10406);
#7570=LINE('',#69887,#10407);
#7571=LINE('',#69891,#10408);
#7572=LINE('',#69894,#10409);
#7573=LINE('',#69895,#10410);
#7574=LINE('',#69900,#10411);
#7575=LINE('',#69902,#10412);
#7576=LINE('',#69903,#10413);
#7577=LINE('',#69908,#10414);
#7578=LINE('',#69909,#10415);
#7579=LINE('',#69920,#10416);
#7580=LINE('',#69928,#10417);
#7581=LINE('',#69932,#10418);
#7582=LINE('',#69933,#10419);
#7583=LINE('',#69936,#10420);
#7584=LINE('',#69944,#10421);
#7585=LINE('',#69949,#10422);
#10126=VECTOR('',#34961,1.55);
#10127=VECTOR('',#34964,10.);
#10128=VECTOR('',#34965,10.);
#10129=VECTOR('',#34966,10.);
#10130=VECTOR('',#34969,10.);
#10131=VECTOR('',#34970,10.);
#10132=VECTOR('',#34973,10.);
#10133=VECTOR('',#34974,10.);
#10134=VECTOR('',#34975,10.);
#10135=VECTOR('',#34978,10.);
#10136=VECTOR('',#34979,10.);
#10137=VECTOR('',#34980,10.);
#10138=VECTOR('',#34983,10.);
#10139=VECTOR('',#34984,10.);
#10140=VECTOR('',#34987,10.);
#10141=VECTOR('',#34988,10.);
#10142=VECTOR('',#34991,10.);
#10143=VECTOR('',#34992,10.);
#10144=VECTOR('',#34993,10.);
#10145=VECTOR('',#34996,10.);
#10146=VECTOR('',#34997,10.);
#10147=VECTOR('',#34998,10.);
#10148=VECTOR('',#35001,10.);
#10149=VECTOR('',#35002,10.);
#10150=VECTOR('',#35005,10.);
#10151=VECTOR('',#35006,10.);
#10152=VECTOR('',#35017,10.);
#10153=VECTOR('',#35018,10.);
#10154=VECTOR('',#35019,10.);
#10155=VECTOR('',#35020,10.);
#10156=VECTOR('',#35025,10.);
#10157=VECTOR('',#35028,10.);
#10158=VECTOR('',#35029,10.);
#10159=VECTOR('',#35036,10.);
#10160=VECTOR('',#35037,10.);
#10161=VECTOR('',#35038,10.);
#10162=VECTOR('',#35039,10.);
#10163=VECTOR('',#35044,10.);
#10164=VECTOR('',#35047,10.);
#10165=VECTOR('',#35048,10.);
#10166=VECTOR('',#35055,10.);
#10167=VECTOR('',#35056,10.);
#10168=VECTOR('',#35057,10.);
#10169=VECTOR('',#35058,10.);
#10170=VECTOR('',#35063,10.);
#10171=VECTOR('',#35066,10.);
#10172=VECTOR('',#35067,10.);
#10173=VECTOR('',#35074,10.);
#10174=VECTOR('',#35075,10.);
#10175=VECTOR('',#35076,10.);
#10176=VECTOR('',#35077,10.);
#10177=VECTOR('',#35082,10.);
#10178=VECTOR('',#35085,10.);
#10179=VECTOR('',#35086,10.);
#10180=VECTOR('',#35093,10.);
#10181=VECTOR('',#35094,10.);
#10182=VECTOR('',#35095,10.);
#10183=VECTOR('',#35096,10.);
#10184=VECTOR('',#35101,10.);
#10185=VECTOR('',#35104,10.);
#10186=VECTOR('',#35105,10.);
#10187=VECTOR('',#35112,10.);
#10188=VECTOR('',#35113,10.);
#10189=VECTOR('',#35114,10.);
#10190=VECTOR('',#35115,10.);
#10191=VECTOR('',#35120,10.);
#10192=VECTOR('',#35123,10.);
#10193=VECTOR('',#35124,10.);
#10194=VECTOR('',#35131,10.);
#10195=VECTOR('',#35132,10.);
#10196=VECTOR('',#35133,10.);
#10197=VECTOR('',#35134,10.);
#10198=VECTOR('',#35139,10.);
#10199=VECTOR('',#35142,10.);
#10200=VECTOR('',#35143,10.);
#10201=VECTOR('',#35150,10.);
#10202=VECTOR('',#35151,10.);
#10203=VECTOR('',#35152,10.);
#10204=VECTOR('',#35153,10.);
#10205=VECTOR('',#35158,10.);
#10206=VECTOR('',#35161,10.);
#10207=VECTOR('',#35162,10.);
#10208=VECTOR('',#35169,10.);
#10209=VECTOR('',#35170,10.);
#10210=VECTOR('',#35171,10.);
#10211=VECTOR('',#35172,10.);
#10212=VECTOR('',#35177,10.);
#10213=VECTOR('',#35180,10.);
#10214=VECTOR('',#35181,10.);
#10215=VECTOR('',#35188,10.);
#10216=VECTOR('',#35189,10.);
#10217=VECTOR('',#35190,10.);
#10218=VECTOR('',#35191,10.);
#10219=VECTOR('',#35196,10.);
#10220=VECTOR('',#35199,10.);
#10221=VECTOR('',#35200,10.);
#10222=VECTOR('',#35207,10.);
#10223=VECTOR('',#35208,10.);
#10224=VECTOR('',#35209,10.);
#10225=VECTOR('',#35210,10.);
#10226=VECTOR('',#35215,10.);
#10227=VECTOR('',#35218,10.);
#10228=VECTOR('',#35219,10.);
#10229=VECTOR('',#35226,10.);
#10230=VECTOR('',#35227,10.);
#10231=VECTOR('',#35228,10.);
#10232=VECTOR('',#35229,10.);
#10233=VECTOR('',#35234,10.);
#10234=VECTOR('',#35237,10.);
#10235=VECTOR('',#35238,10.);
#10236=VECTOR('',#35245,10.);
#10237=VECTOR('',#35246,10.);
#10238=VECTOR('',#35247,10.);
#10239=VECTOR('',#35248,10.);
#10240=VECTOR('',#35253,10.);
#10241=VECTOR('',#35256,10.);
#10242=VECTOR('',#35257,10.);
#10243=VECTOR('',#35264,10.);
#10244=VECTOR('',#35265,10.);
#10245=VECTOR('',#35266,10.);
#10246=VECTOR('',#35267,10.);
#10247=VECTOR('',#35272,10.);
#10248=VECTOR('',#35275,10.);
#10249=VECTOR('',#35276,10.);
#10250=VECTOR('',#35283,10.);
#10251=VECTOR('',#35284,10.);
#10252=VECTOR('',#35285,10.);
#10253=VECTOR('',#35286,10.);
#10254=VECTOR('',#35291,10.);
#10255=VECTOR('',#35294,10.);
#10256=VECTOR('',#35295,10.);
#10257=VECTOR('',#35302,10.);
#10258=VECTOR('',#35303,10.);
#10259=VECTOR('',#35304,10.);
#10260=VECTOR('',#35305,10.);
#10261=VECTOR('',#35310,10.);
#10262=VECTOR('',#35313,10.);
#10263=VECTOR('',#35314,10.);
#10264=VECTOR('',#35321,10.);
#10265=VECTOR('',#35322,10.);
#10266=VECTOR('',#35323,10.);
#10267=VECTOR('',#35324,10.);
#10268=VECTOR('',#35329,10.);
#10269=VECTOR('',#35332,10.);
#10270=VECTOR('',#35333,10.);
#10271=VECTOR('',#35340,10.);
#10272=VECTOR('',#35341,10.);
#10273=VECTOR('',#35342,10.);
#10274=VECTOR('',#35343,10.);
#10275=VECTOR('',#35348,10.);
#10276=VECTOR('',#35351,10.);
#10277=VECTOR('',#35352,10.);
#10278=VECTOR('',#35359,10.);
#10279=VECTOR('',#35360,10.);
#10280=VECTOR('',#35361,10.);
#10281=VECTOR('',#35362,10.);
#10282=VECTOR('',#35367,10.);
#10283=VECTOR('',#35372,10.);
#10284=VECTOR('',#35373,10.);
#10285=VECTOR('',#35382,10.);
#10286=VECTOR('',#35383,10.);
#10287=VECTOR('',#35384,10.);
#10288=VECTOR('',#35385,10.);
#10289=VECTOR('',#35390,10.);
#10290=VECTOR('',#35393,10.);
#10291=VECTOR('',#35394,10.);
#10292=VECTOR('',#35401,10.);
#10293=VECTOR('',#35402,10.);
#10294=VECTOR('',#35403,10.);
#10295=VECTOR('',#35404,10.);
#10296=VECTOR('',#35409,10.);
#10297=VECTOR('',#35412,10.);
#10298=VECTOR('',#35413,10.);
#10299=VECTOR('',#35420,10.);
#10300=VECTOR('',#35421,10.);
#10301=VECTOR('',#35422,10.);
#10302=VECTOR('',#35423,10.);
#10303=VECTOR('',#35428,10.);
#10304=VECTOR('',#35431,10.);
#10305=VECTOR('',#35432,10.);
#10306=VECTOR('',#35439,10.);
#10307=VECTOR('',#35440,10.);
#10308=VECTOR('',#35441,10.);
#10309=VECTOR('',#35442,10.);
#10310=VECTOR('',#35447,10.);
#10311=VECTOR('',#35450,10.);
#10312=VECTOR('',#35451,10.);
#10313=VECTOR('',#35458,10.);
#10314=VECTOR('',#35459,10.);
#10315=VECTOR('',#35460,10.);
#10316=VECTOR('',#35461,10.);
#10317=VECTOR('',#35466,10.);
#10318=VECTOR('',#35469,10.);
#10319=VECTOR('',#35470,10.);
#10320=VECTOR('',#35477,10.);
#10321=VECTOR('',#35478,10.);
#10322=VECTOR('',#35479,10.);
#10323=VECTOR('',#35480,10.);
#10324=VECTOR('',#35485,10.);
#10325=VECTOR('',#35488,10.);
#10326=VECTOR('',#35489,10.);
#10327=VECTOR('',#35496,10.);
#10328=VECTOR('',#35497,10.);
#10329=VECTOR('',#35498,10.);
#10330=VECTOR('',#35499,10.);
#10331=VECTOR('',#35504,10.);
#10332=VECTOR('',#35507,10.);
#10333=VECTOR('',#35508,10.);
#10334=VECTOR('',#35515,10.);
#10335=VECTOR('',#35516,10.);
#10336=VECTOR('',#35517,10.);
#10337=VECTOR('',#35518,10.);
#10338=VECTOR('',#35523,10.);
#10339=VECTOR('',#35526,10.);
#10340=VECTOR('',#35527,10.);
#10341=VECTOR('',#35534,10.);
#10342=VECTOR('',#35535,10.);
#10343=VECTOR('',#35536,10.);
#10344=VECTOR('',#35537,10.);
#10345=VECTOR('',#35542,10.);
#10346=VECTOR('',#35545,10.);
#10347=VECTOR('',#35546,10.);
#10348=VECTOR('',#35553,10.);
#10349=VECTOR('',#35554,10.);
#10350=VECTOR('',#35555,10.);
#10351=VECTOR('',#35556,10.);
#10352=VECTOR('',#35561,10.);
#10353=VECTOR('',#35564,10.);
#10354=VECTOR('',#35565,10.);
#10355=VECTOR('',#35572,10.);
#10356=VECTOR('',#35573,10.);
#10357=VECTOR('',#35574,10.);
#10358=VECTOR('',#35575,10.);
#10359=VECTOR('',#35580,10.);
#10360=VECTOR('',#35583,10.);
#10361=VECTOR('',#35584,10.);
#10362=VECTOR('',#35591,10.);
#10363=VECTOR('',#35592,10.);
#10364=VECTOR('',#35593,10.);
#10365=VECTOR('',#35594,10.);
#10366=VECTOR('',#35599,10.);
#10367=VECTOR('',#35602,10.);
#10368=VECTOR('',#35603,10.);
#10369=VECTOR('',#35610,10.);
#10370=VECTOR('',#35611,10.);
#10371=VECTOR('',#35612,10.);
#10372=VECTOR('',#35613,10.);
#10373=VECTOR('',#35618,10.);
#10374=VECTOR('',#35621,10.);
#10375=VECTOR('',#35622,10.);
#10376=VECTOR('',#35629,10.);
#10377=VECTOR('',#35630,10.);
#10378=VECTOR('',#35631,10.);
#10379=VECTOR('',#35632,10.);
#10380=VECTOR('',#35637,10.);
#10381=VECTOR('',#35640,10.);
#10382=VECTOR('',#35641,10.);
#10383=VECTOR('',#35648,10.);
#10384=VECTOR('',#35649,10.);
#10385=VECTOR('',#35650,10.);
#10386=VECTOR('',#35651,10.);
#10387=VECTOR('',#35656,10.);
#10388=VECTOR('',#35659,10.);
#10389=VECTOR('',#35660,10.);
#10390=VECTOR('',#35667,10.);
#10391=VECTOR('',#35668,10.);
#10392=VECTOR('',#35669,10.);
#10393=VECTOR('',#35670,10.);
#10394=VECTOR('',#35675,10.);
#10395=VECTOR('',#35678,10.);
#10396=VECTOR('',#35679,10.);
#10397=VECTOR('',#35686,10.);
#10398=VECTOR('',#35687,10.);
#10399=VECTOR('',#35688,10.);
#10400=VECTOR('',#35689,10.);
#10401=VECTOR('',#35694,10.);
#10402=VECTOR('',#35697,10.);
#10403=VECTOR('',#35698,10.);
#10404=VECTOR('',#35705,10.);
#10405=VECTOR('',#35706,10.);
#10406=VECTOR('',#35707,10.);
#10407=VECTOR('',#35708,10.);
#10408=VECTOR('',#35713,10.);
#10409=VECTOR('',#35716,10.);
#10410=VECTOR('',#35717,10.);
#10411=VECTOR('',#35724,10.);
#10412=VECTOR('',#35725,10.);
#10413=VECTOR('',#35726,10.);
#10414=VECTOR('',#35733,10.);
#10415=VECTOR('',#35734,10.);
#10416=VECTOR('',#35751,3.905);
#10417=VECTOR('',#35762,7.2);
#10418=VECTOR('',#35767,7.5);
#10419=VECTOR('',#35768,7.5);
#10420=VECTOR('',#35771,7.3);
#10421=VECTOR('',#35782,2.8);
#10422=VECTOR('',#35789,2.01);
#12825=CIRCLE('',#32502,7.5);
#12826=CIRCLE('',#32504,7.5);
#12827=CIRCLE('',#32507,7.5);
#12828=CIRCLE('',#32510,7.5);
#12829=CIRCLE('',#32513,7.5);
#12830=CIRCLE('',#32516,7.5);
#12831=CIRCLE('',#32519,7.5);
#12832=CIRCLE('',#32522,7.5);
#12833=CIRCLE('',#32525,7.5);
#12834=CIRCLE('',#32528,7.5);
#12835=CIRCLE('',#32531,7.5);
#12836=CIRCLE('',#32534,7.5);
#12837=CIRCLE('',#32537,7.5);
#12838=CIRCLE('',#32540,7.5);
#12839=CIRCLE('',#32543,7.5);
#12840=CIRCLE('',#32546,7.5);
#12841=CIRCLE('',#32549,7.5);
#12842=CIRCLE('',#32552,7.5);
#12843=CIRCLE('',#32555,7.5);
#12844=CIRCLE('',#32558,7.5);
#12845=CIRCLE('',#32561,7.5);
#12846=CIRCLE('',#32564,7.5);
#12847=CIRCLE('',#32567,7.5);
#12848=CIRCLE('',#32570,7.5);
#12849=CIRCLE('',#32573,7.5);
#12850=CIRCLE('',#32576,7.5);
#12851=CIRCLE('',#32579,7.5);
#12852=CIRCLE('',#32582,7.5);
#12853=CIRCLE('',#32585,7.5);
#12854=CIRCLE('',#32588,7.5);
#12855=CIRCLE('',#32591,7.5);
#12856=CIRCLE('',#32594,7.5);
#12857=CIRCLE('',#32597,7.5);
#12858=CIRCLE('',#32600,7.5);
#12859=CIRCLE('',#32603,7.5);
#12860=CIRCLE('',#32606,7.5);
#12861=CIRCLE('',#32609,7.5);
#12862=CIRCLE('',#32612,7.5);
#12863=CIRCLE('',#32615,7.5);
#12864=CIRCLE('',#32616,7.5);
#12865=CIRCLE('',#32619,7.5);
#12866=CIRCLE('',#32620,7.5);
#12867=CIRCLE('',#32623,7.5);
#12868=CIRCLE('',#32626,7.5);
#12869=CIRCLE('',#32629,7.5);
#12870=CIRCLE('',#32632,7.5);
#12871=CIRCLE('',#32635,7.5);
#12872=CIRCLE('',#32638,7.5);
#12873=CIRCLE('',#32641,7.5);
#12874=CIRCLE('',#32644,7.5);
#12875=CIRCLE('',#32647,7.5);
#12876=CIRCLE('',#32650,7.5);
#12877=CIRCLE('',#32653,7.5);
#12878=CIRCLE('',#32656,7.5);
#12879=CIRCLE('',#32659,7.5);
#12880=CIRCLE('',#32662,7.5);
#12881=CIRCLE('',#32665,7.5);
#12882=CIRCLE('',#32668,7.5);
#12883=CIRCLE('',#32671,7.5);
#12884=CIRCLE('',#32674,7.5);
#12885=CIRCLE('',#32677,7.5);
#12886=CIRCLE('',#32680,7.5);
#12887=CIRCLE('',#32683,7.5);
#12888=CIRCLE('',#32686,7.5);
#12889=CIRCLE('',#32689,7.5);
#12890=CIRCLE('',#32692,7.5);
#12891=CIRCLE('',#32695,7.5);
#12892=CIRCLE('',#32698,7.5);
#12893=CIRCLE('',#32701,7.5);
#12894=CIRCLE('',#32704,7.5);
#12895=CIRCLE('',#32707,7.5);
#12896=CIRCLE('',#32710,7.5);
#12897=CIRCLE('',#32713,7.5);
#12898=CIRCLE('',#32716,7.5);
#12899=CIRCLE('',#32719,7.5);
#12900=CIRCLE('',#32722,7.5);
#12901=CIRCLE('',#32725,7.5);
#12902=CIRCLE('',#32728,7.5);
#12903=CIRCLE('',#32731,7.5);
#12904=CIRCLE('',#32734,7.5);
#12905=CIRCLE('',#32736,7.5);
#12906=CIRCLE('',#32738,7.5);
#12907=CIRCLE('',#32740,2.01);
#12908=CIRCLE('',#32741,5.8);
#12909=CIRCLE('',#32743,6.9);
#12910=CIRCLE('',#32745,7.5);
#12911=CIRCLE('',#32747,7.5);
#12912=CIRCLE('',#32749,7.1);
#12913=CIRCLE('',#32751,2.8);
#12914=CIRCLE('',#32753,2.8);
#12915=CIRCLE('',#32755,2.01);
#13577=VERTEX_POINT('',#69012);
#13578=VERTEX_POINT('',#69013);
#13579=VERTEX_POINT('',#69020);
#13580=VERTEX_POINT('',#69022);
#13581=VERTEX_POINT('',#69024);
#13582=VERTEX_POINT('',#69031);
#13583=VERTEX_POINT('',#69033);
#13584=VERTEX_POINT('',#69035);
#13585=VERTEX_POINT('',#69042);
#13586=VERTEX_POINT('',#69044);
#13587=VERTEX_POINT('',#69046);
#13588=VERTEX_POINT('',#69058);
#13589=VERTEX_POINT('',#69060);
#13590=VERTEX_POINT('',#69062);
#13591=VERTEX_POINT('',#69069);
#13592=VERTEX_POINT('',#69071);
#13593=VERTEX_POINT('',#69073);
#13594=VERTEX_POINT('',#69080);
#13595=VERTEX_POINT('',#69082);
#13596=VERTEX_POINT('',#69090);
#13597=VERTEX_POINT('',#69092);
#13598=VERTEX_POINT('',#69138);
#13599=VERTEX_POINT('',#69140);
#13600=VERTEX_POINT('',#69144);
#13601=VERTEX_POINT('',#69148);
#13602=VERTEX_POINT('',#69150);
#13603=VERTEX_POINT('',#69154);
#13604=VERTEX_POINT('',#69156);
#13605=VERTEX_POINT('',#69160);
#13606=VERTEX_POINT('',#69164);
#13607=VERTEX_POINT('',#69168);
#13608=VERTEX_POINT('',#69170);
#13609=VERTEX_POINT('',#69174);
#13610=VERTEX_POINT('',#69176);
#13611=VERTEX_POINT('',#69180);
#13612=VERTEX_POINT('',#69184);
#13613=VERTEX_POINT('',#69192);
#13614=VERTEX_POINT('',#69193);
#13615=VERTEX_POINT('',#69195);
#13616=VERTEX_POINT('',#69197);
#13617=VERTEX_POINT('',#69201);
#13618=VERTEX_POINT('',#69205);
#13619=VERTEX_POINT('',#69211);
#13620=VERTEX_POINT('',#69212);
#13621=VERTEX_POINT('',#69214);
#13622=VERTEX_POINT('',#69216);
#13623=VERTEX_POINT('',#69220);
#13624=VERTEX_POINT('',#69224);
#13625=VERTEX_POINT('',#69230);
#13626=VERTEX_POINT('',#69231);
#13627=VERTEX_POINT('',#69233);
#13628=VERTEX_POINT('',#69235);
#13629=VERTEX_POINT('',#69239);
#13630=VERTEX_POINT('',#69243);
#13631=VERTEX_POINT('',#69249);
#13632=VERTEX_POINT('',#69250);
#13633=VERTEX_POINT('',#69252);
#13634=VERTEX_POINT('',#69254);
#13635=VERTEX_POINT('',#69258);
#13636=VERTEX_POINT('',#69262);
#13637=VERTEX_POINT('',#69268);
#13638=VERTEX_POINT('',#69269);
#13639=VERTEX_POINT('',#69271);
#13640=VERTEX_POINT('',#69273);
#13641=VERTEX_POINT('',#69277);
#13642=VERTEX_POINT('',#69281);
#13643=VERTEX_POINT('',#69287);
#13644=VERTEX_POINT('',#69288);
#13645=VERTEX_POINT('',#69290);
#13646=VERTEX_POINT('',#69292);
#13647=VERTEX_POINT('',#69296);
#13648=VERTEX_POINT('',#69300);
#13649=VERTEX_POINT('',#69306);
#13650=VERTEX_POINT('',#69307);
#13651=VERTEX_POINT('',#69309);
#13652=VERTEX_POINT('',#69311);
#13653=VERTEX_POINT('',#69315);
#13654=VERTEX_POINT('',#69319);
#13655=VERTEX_POINT('',#69325);
#13656=VERTEX_POINT('',#69326);
#13657=VERTEX_POINT('',#69328);
#13658=VERTEX_POINT('',#69330);
#13659=VERTEX_POINT('',#69334);
#13660=VERTEX_POINT('',#69338);
#13661=VERTEX_POINT('',#69344);
#13662=VERTEX_POINT('',#69345);
#13663=VERTEX_POINT('',#69347);
#13664=VERTEX_POINT('',#69349);
#13665=VERTEX_POINT('',#69353);
#13666=VERTEX_POINT('',#69357);
#13667=VERTEX_POINT('',#69363);
#13668=VERTEX_POINT('',#69364);
#13669=VERTEX_POINT('',#69366);
#13670=VERTEX_POINT('',#69368);
#13671=VERTEX_POINT('',#69372);
#13672=VERTEX_POINT('',#69376);
#13673=VERTEX_POINT('',#69382);
#13674=VERTEX_POINT('',#69383);
#13675=VERTEX_POINT('',#69385);
#13676=VERTEX_POINT('',#69387);
#13677=VERTEX_POINT('',#69391);
#13678=VERTEX_POINT('',#69395);
#13679=VERTEX_POINT('',#69401);
#13680=VERTEX_POINT('',#69402);
#13681=VERTEX_POINT('',#69404);
#13682=VERTEX_POINT('',#69406);
#13683=VERTEX_POINT('',#69410);
#13684=VERTEX_POINT('',#69414);
#13685=VERTEX_POINT('',#69420);
#13686=VERTEX_POINT('',#69421);
#13687=VERTEX_POINT('',#69423);
#13688=VERTEX_POINT('',#69425);
#13689=VERTEX_POINT('',#69429);
#13690=VERTEX_POINT('',#69433);
#13691=VERTEX_POINT('',#69439);
#13692=VERTEX_POINT('',#69440);
#13693=VERTEX_POINT('',#69442);
#13694=VERTEX_POINT('',#69444);
#13695=VERTEX_POINT('',#69448);
#13696=VERTEX_POINT('',#69452);
#13697=VERTEX_POINT('',#69458);
#13698=VERTEX_POINT('',#69459);
#13699=VERTEX_POINT('',#69461);
#13700=VERTEX_POINT('',#69463);
#13701=VERTEX_POINT('',#69467);
#13702=VERTEX_POINT('',#69471);
#13703=VERTEX_POINT('',#69477);
#13704=VERTEX_POINT('',#69478);
#13705=VERTEX_POINT('',#69480);
#13706=VERTEX_POINT('',#69482);
#13707=VERTEX_POINT('',#69486);
#13708=VERTEX_POINT('',#69490);
#13709=VERTEX_POINT('',#69496);
#13710=VERTEX_POINT('',#69497);
#13711=VERTEX_POINT('',#69499);
#13712=VERTEX_POINT('',#69501);
#13713=VERTEX_POINT('',#69505);
#13714=VERTEX_POINT('',#69509);
#13715=VERTEX_POINT('',#69515);
#13716=VERTEX_POINT('',#69516);
#13717=VERTEX_POINT('',#69518);
#13718=VERTEX_POINT('',#69520);
#13719=VERTEX_POINT('',#69524);
#13720=VERTEX_POINT('',#69528);
#13721=VERTEX_POINT('',#69534);
#13722=VERTEX_POINT('',#69535);
#13723=VERTEX_POINT('',#69537);
#13724=VERTEX_POINT('',#69539);
#13725=VERTEX_POINT('',#69543);
#13726=VERTEX_POINT('',#69545);
#13727=VERTEX_POINT('',#69549);
#13728=VERTEX_POINT('',#69553);
#13729=VERTEX_POINT('',#69557);
#13730=VERTEX_POINT('',#69558);
#13731=VERTEX_POINT('',#69560);
#13732=VERTEX_POINT('',#69562);
#13733=VERTEX_POINT('',#69566);
#13734=VERTEX_POINT('',#69570);
#13735=VERTEX_POINT('',#69576);
#13736=VERTEX_POINT('',#69577);
#13737=VERTEX_POINT('',#69579);
#13738=VERTEX_POINT('',#69581);
#13739=VERTEX_POINT('',#69585);
#13740=VERTEX_POINT('',#69589);
#13741=VERTEX_POINT('',#69595);
#13742=VERTEX_POINT('',#69596);
#13743=VERTEX_POINT('',#69598);
#13744=VERTEX_POINT('',#69600);
#13745=VERTEX_POINT('',#69604);
#13746=VERTEX_POINT('',#69608);
#13747=VERTEX_POINT('',#69614);
#13748=VERTEX_POINT('',#69615);
#13749=VERTEX_POINT('',#69617);
#13750=VERTEX_POINT('',#69619);
#13751=VERTEX_POINT('',#69623);
#13752=VERTEX_POINT('',#69627);
#13753=VERTEX_POINT('',#69633);
#13754=VERTEX_POINT('',#69634);
#13755=VERTEX_POINT('',#69636);
#13756=VERTEX_POINT('',#69638);
#13757=VERTEX_POINT('',#69642);
#13758=VERTEX_POINT('',#69646);
#13759=VERTEX_POINT('',#69652);
#13760=VERTEX_POINT('',#69653);
#13761=VERTEX_POINT('',#69655);
#13762=VERTEX_POINT('',#69657);
#13763=VERTEX_POINT('',#69661);
#13764=VERTEX_POINT('',#69665);
#13765=VERTEX_POINT('',#69671);
#13766=VERTEX_POINT('',#69672);
#13767=VERTEX_POINT('',#69674);
#13768=VERTEX_POINT('',#69676);
#13769=VERTEX_POINT('',#69680);
#13770=VERTEX_POINT('',#69684);
#13771=VERTEX_POINT('',#69690);
#13772=VERTEX_POINT('',#69691);
#13773=VERTEX_POINT('',#69693);
#13774=VERTEX_POINT('',#69695);
#13775=VERTEX_POINT('',#69699);
#13776=VERTEX_POINT('',#69703);
#13777=VERTEX_POINT('',#69709);
#13778=VERTEX_POINT('',#69710);
#13779=VERTEX_POINT('',#69712);
#13780=VERTEX_POINT('',#69714);
#13781=VERTEX_POINT('',#69718);
#13782=VERTEX_POINT('',#69722);
#13783=VERTEX_POINT('',#69728);
#13784=VERTEX_POINT('',#69729);
#13785=VERTEX_POINT('',#69731);
#13786=VERTEX_POINT('',#69733);
#13787=VERTEX_POINT('',#69737);
#13788=VERTEX_POINT('',#69741);
#13789=VERTEX_POINT('',#69747);
#13790=VERTEX_POINT('',#69748);
#13791=VERTEX_POINT('',#69750);
#13792=VERTEX_POINT('',#69752);
#13793=VERTEX_POINT('',#69756);
#13794=VERTEX_POINT('',#69760);
#13795=VERTEX_POINT('',#69766);
#13796=VERTEX_POINT('',#69767);
#13797=VERTEX_POINT('',#69769);
#13798=VERTEX_POINT('',#69771);
#13799=VERTEX_POINT('',#69775);
#13800=VERTEX_POINT('',#69779);
#13801=VERTEX_POINT('',#69785);
#13802=VERTEX_POINT('',#69786);
#13803=VERTEX_POINT('',#69788);
#13804=VERTEX_POINT('',#69790);
#13805=VERTEX_POINT('',#69794);
#13806=VERTEX_POINT('',#69798);
#13807=VERTEX_POINT('',#69804);
#13808=VERTEX_POINT('',#69805);
#13809=VERTEX_POINT('',#69807);
#13810=VERTEX_POINT('',#69809);
#13811=VERTEX_POINT('',#69813);
#13812=VERTEX_POINT('',#69817);
#13813=VERTEX_POINT('',#69823);
#13814=VERTEX_POINT('',#69824);
#13815=VERTEX_POINT('',#69826);
#13816=VERTEX_POINT('',#69828);
#13817=VERTEX_POINT('',#69832);
#13818=VERTEX_POINT('',#69836);
#13819=VERTEX_POINT('',#69842);
#13820=VERTEX_POINT('',#69843);
#13821=VERTEX_POINT('',#69845);
#13822=VERTEX_POINT('',#69847);
#13823=VERTEX_POINT('',#69851);
#13824=VERTEX_POINT('',#69855);
#13825=VERTEX_POINT('',#69861);
#13826=VERTEX_POINT('',#69862);
#13827=VERTEX_POINT('',#69864);
#13828=VERTEX_POINT('',#69866);
#13829=VERTEX_POINT('',#69870);
#13830=VERTEX_POINT('',#69874);
#13831=VERTEX_POINT('',#69880);
#13832=VERTEX_POINT('',#69881);
#13833=VERTEX_POINT('',#69883);
#13834=VERTEX_POINT('',#69885);
#13835=VERTEX_POINT('',#69889);
#13836=VERTEX_POINT('',#69893);
#13837=VERTEX_POINT('',#69899);
#13838=VERTEX_POINT('',#69901);
#13839=VERTEX_POINT('',#69907);
#13840=VERTEX_POINT('',#69917);
#13841=VERTEX_POINT('',#69919);
#13842=VERTEX_POINT('',#69923);
#13843=VERTEX_POINT('',#69926);
#13844=VERTEX_POINT('',#69930);
#13845=VERTEX_POINT('',#69935);
#13846=VERTEX_POINT('',#69939);
#13847=VERTEX_POINT('',#69942);
#13848=VERTEX_POINT('',#69946);
#16833=EDGE_CURVE('',#13577,#13578,#811,.T.);
#16834=EDGE_CURVE('',#13579,#13577,#288,.T.);
#16835=EDGE_CURVE('',#13580,#13579,#289,.T.);
#16836=EDGE_CURVE('',#13581,#13580,#812,.T.);
#16837=EDGE_CURVE('',#13582,#13581,#290,.T.);
#16838=EDGE_CURVE('',#13583,#13582,#291,.T.);
#16839=EDGE_CURVE('',#13584,#13583,#813,.T.);
#16840=EDGE_CURVE('',#13585,#13584,#292,.T.);
#16841=EDGE_CURVE('',#13586,#13585,#293,.T.);
#16842=EDGE_CURVE('',#13587,#13586,#814,.T.);
#16843=EDGE_CURVE('',#13588,#13587,#294,.T.);
#16844=EDGE_CURVE('',#13589,#13588,#295,.T.);
#16845=EDGE_CURVE('',#13590,#13589,#815,.T.);
#16846=EDGE_CURVE('',#13591,#13590,#296,.T.);
#16847=EDGE_CURVE('',#13592,#13591,#297,.T.);
#16848=EDGE_CURVE('',#13593,#13592,#816,.T.);
#16849=EDGE_CURVE('',#13594,#13593,#298,.T.);
#16850=EDGE_CURVE('',#13595,#13594,#299,.T.);
#16851=EDGE_CURVE('',#13578,#13595,#817,.T.);
#16852=EDGE_CURVE('',#13578,#13596,#7289,.T.);
#16853=EDGE_CURVE('',#13597,#13596,#818,.T.);
#16854=EDGE_CURVE('',#13596,#13597,#819,.T.);
#16855=EDGE_CURVE('',#13598,#13577,#7290,.T.);
#16856=EDGE_CURVE('',#13598,#13599,#7291,.T.);
#16857=EDGE_CURVE('',#13599,#13579,#7292,.T.);
#16858=EDGE_CURVE('',#13599,#13600,#7293,.T.);
#16859=EDGE_CURVE('',#13580,#13600,#7294,.T.);
#16860=EDGE_CURVE('',#13601,#13585,#7295,.T.);
#16861=EDGE_CURVE('',#13601,#13602,#7296,.T.);
#16862=EDGE_CURVE('',#13586,#13602,#7297,.T.);
#16863=EDGE_CURVE('',#13603,#13587,#7298,.T.);
#16864=EDGE_CURVE('',#13603,#13604,#7299,.T.);
#16865=EDGE_CURVE('',#13588,#13604,#7300,.T.);
#16866=EDGE_CURVE('',#13605,#13584,#7301,.T.);
#16867=EDGE_CURVE('',#13605,#13601,#7302,.T.);
#16868=EDGE_CURVE('',#13604,#13606,#7303,.T.);
#16869=EDGE_CURVE('',#13589,#13606,#7304,.T.);
#16870=EDGE_CURVE('',#13607,#13581,#7305,.T.);
#16871=EDGE_CURVE('',#13607,#13608,#7306,.T.);
#16872=EDGE_CURVE('',#13608,#13582,#7307,.T.);
#16873=EDGE_CURVE('',#13591,#13609,#7308,.T.);
#16874=EDGE_CURVE('',#13609,#13610,#7309,.T.);
#16875=EDGE_CURVE('',#13592,#13610,#7310,.T.);
#16876=EDGE_CURVE('',#13608,#13611,#7311,.T.);
#16877=EDGE_CURVE('',#13583,#13611,#7312,.T.);
#16878=EDGE_CURVE('',#13612,#13590,#7313,.T.);
#16879=EDGE_CURVE('',#13612,#13609,#7314,.T.);
#16880=EDGE_CURVE('',#13602,#13605,#12825,.T.);
#16881=EDGE_CURVE('',#13606,#13603,#12826,.T.);
#16882=EDGE_CURVE('',#13613,#13614,#7315,.T.);
#16883=EDGE_CURVE('',#13613,#13615,#7316,.T.);
#16884=EDGE_CURVE('',#13616,#13615,#7317,.T.);
#16885=EDGE_CURVE('',#13616,#13614,#7318,.T.);
#16886=EDGE_CURVE('',#13614,#13617,#12827,.T.);
#16887=EDGE_CURVE('',#13617,#13616,#7319,.T.);
#16888=EDGE_CURVE('',#13617,#13618,#7320,.T.);
#16889=EDGE_CURVE('',#13615,#13618,#7321,.T.);
#16890=EDGE_CURVE('',#13618,#13613,#12828,.T.);
#16891=EDGE_CURVE('',#13619,#13620,#7322,.T.);
#16892=EDGE_CURVE('',#13619,#13621,#7323,.T.);
#16893=EDGE_CURVE('',#13622,#13621,#7324,.T.);
#16894=EDGE_CURVE('',#13622,#13620,#7325,.T.);
#16895=EDGE_CURVE('',#13620,#13623,#12829,.T.);
#16896=EDGE_CURVE('',#13623,#13622,#7326,.T.);
#16897=EDGE_CURVE('',#13623,#13624,#7327,.T.);
#16898=EDGE_CURVE('',#13621,#13624,#7328,.T.);
#16899=EDGE_CURVE('',#13624,#13619,#12830,.T.);
#16900=EDGE_CURVE('',#13625,#13626,#7329,.T.);
#16901=EDGE_CURVE('',#13625,#13627,#7330,.T.);
#16902=EDGE_CURVE('',#13628,#13627,#7331,.T.);
#16903=EDGE_CURVE('',#13628,#13626,#7332,.T.);
#16904=EDGE_CURVE('',#13626,#13629,#12831,.T.);
#16905=EDGE_CURVE('',#13629,#13628,#7333,.T.);
#16906=EDGE_CURVE('',#13629,#13630,#7334,.T.);
#16907=EDGE_CURVE('',#13627,#13630,#7335,.T.);
#16908=EDGE_CURVE('',#13630,#13625,#12832,.T.);
#16909=EDGE_CURVE('',#13631,#13632,#7336,.T.);
#16910=EDGE_CURVE('',#13631,#13633,#7337,.T.);
#16911=EDGE_CURVE('',#13634,#13633,#7338,.T.);
#16912=EDGE_CURVE('',#13634,#13632,#7339,.T.);
#16913=EDGE_CURVE('',#13632,#13635,#12833,.T.);
#16914=EDGE_CURVE('',#13635,#13634,#7340,.T.);
#16915=EDGE_CURVE('',#13635,#13636,#7341,.T.);
#16916=EDGE_CURVE('',#13633,#13636,#7342,.T.);
#16917=EDGE_CURVE('',#13636,#13631,#12834,.T.);
#16918=EDGE_CURVE('',#13637,#13638,#7343,.T.);
#16919=EDGE_CURVE('',#13637,#13639,#7344,.T.);
#16920=EDGE_CURVE('',#13640,#13639,#7345,.T.);
#16921=EDGE_CURVE('',#13640,#13638,#7346,.T.);
#16922=EDGE_CURVE('',#13638,#13641,#12835,.T.);
#16923=EDGE_CURVE('',#13641,#13640,#7347,.T.);
#16924=EDGE_CURVE('',#13641,#13642,#7348,.T.);
#16925=EDGE_CURVE('',#13639,#13642,#7349,.T.);
#16926=EDGE_CURVE('',#13642,#13637,#12836,.T.);
#16927=EDGE_CURVE('',#13643,#13644,#7350,.T.);
#16928=EDGE_CURVE('',#13643,#13645,#7351,.T.);
#16929=EDGE_CURVE('',#13646,#13645,#7352,.T.);
#16930=EDGE_CURVE('',#13646,#13644,#7353,.T.);
#16931=EDGE_CURVE('',#13644,#13647,#12837,.T.);
#16932=EDGE_CURVE('',#13647,#13646,#7354,.T.);
#16933=EDGE_CURVE('',#13647,#13648,#7355,.T.);
#16934=EDGE_CURVE('',#13645,#13648,#7356,.T.);
#16935=EDGE_CURVE('',#13648,#13643,#12838,.T.);
#16936=EDGE_CURVE('',#13649,#13650,#7357,.T.);
#16937=EDGE_CURVE('',#13649,#13651,#7358,.T.);
#16938=EDGE_CURVE('',#13652,#13651,#7359,.T.);
#16939=EDGE_CURVE('',#13652,#13650,#7360,.T.);
#16940=EDGE_CURVE('',#13650,#13653,#12839,.T.);
#16941=EDGE_CURVE('',#13653,#13652,#7361,.T.);
#16942=EDGE_CURVE('',#13653,#13654,#7362,.T.);
#16943=EDGE_CURVE('',#13651,#13654,#7363,.T.);
#16944=EDGE_CURVE('',#13654,#13649,#12840,.T.);
#16945=EDGE_CURVE('',#13655,#13656,#7364,.T.);
#16946=EDGE_CURVE('',#13655,#13657,#7365,.T.);
#16947=EDGE_CURVE('',#13658,#13657,#7366,.T.);
#16948=EDGE_CURVE('',#13658,#13656,#7367,.T.);
#16949=EDGE_CURVE('',#13656,#13659,#12841,.T.);
#16950=EDGE_CURVE('',#13659,#13658,#7368,.T.);
#16951=EDGE_CURVE('',#13659,#13660,#7369,.T.);
#16952=EDGE_CURVE('',#13657,#13660,#7370,.T.);
#16953=EDGE_CURVE('',#13660,#13655,#12842,.T.);
#16954=EDGE_CURVE('',#13661,#13662,#7371,.T.);
#16955=EDGE_CURVE('',#13661,#13663,#7372,.T.);
#16956=EDGE_CURVE('',#13664,#13663,#7373,.T.);
#16957=EDGE_CURVE('',#13664,#13662,#7374,.T.);
#16958=EDGE_CURVE('',#13662,#13665,#12843,.T.);
#16959=EDGE_CURVE('',#13665,#13664,#7375,.T.);
#16960=EDGE_CURVE('',#13665,#13666,#7376,.T.);
#16961=EDGE_CURVE('',#13663,#13666,#7377,.T.);
#16962=EDGE_CURVE('',#13666,#13661,#12844,.T.);
#16963=EDGE_CURVE('',#13667,#13668,#7378,.T.);
#16964=EDGE_CURVE('',#13667,#13669,#7379,.T.);
#16965=EDGE_CURVE('',#13670,#13669,#7380,.T.);
#16966=EDGE_CURVE('',#13670,#13668,#7381,.T.);
#16967=EDGE_CURVE('',#13668,#13671,#12845,.T.);
#16968=EDGE_CURVE('',#13671,#13670,#7382,.T.);
#16969=EDGE_CURVE('',#13671,#13672,#7383,.T.);
#16970=EDGE_CURVE('',#13669,#13672,#7384,.T.);
#16971=EDGE_CURVE('',#13672,#13667,#12846,.T.);
#16972=EDGE_CURVE('',#13673,#13674,#7385,.T.);
#16973=EDGE_CURVE('',#13673,#13675,#7386,.T.);
#16974=EDGE_CURVE('',#13676,#13675,#7387,.T.);
#16975=EDGE_CURVE('',#13676,#13674,#7388,.T.);
#16976=EDGE_CURVE('',#13674,#13677,#12847,.T.);
#16977=EDGE_CURVE('',#13677,#13676,#7389,.T.);
#16978=EDGE_CURVE('',#13677,#13678,#7390,.T.);
#16979=EDGE_CURVE('',#13675,#13678,#7391,.T.);
#16980=EDGE_CURVE('',#13678,#13673,#12848,.T.);
#16981=EDGE_CURVE('',#13679,#13680,#7392,.T.);
#16982=EDGE_CURVE('',#13679,#13681,#7393,.T.);
#16983=EDGE_CURVE('',#13682,#13681,#7394,.T.);
#16984=EDGE_CURVE('',#13682,#13680,#7395,.T.);
#16985=EDGE_CURVE('',#13680,#13683,#12849,.T.);
#16986=EDGE_CURVE('',#13683,#13682,#7396,.T.);
#16987=EDGE_CURVE('',#13683,#13684,#7397,.T.);
#16988=EDGE_CURVE('',#13681,#13684,#7398,.T.);
#16989=EDGE_CURVE('',#13684,#13679,#12850,.T.);
#16990=EDGE_CURVE('',#13685,#13686,#7399,.T.);
#16991=EDGE_CURVE('',#13685,#13687,#7400,.T.);
#16992=EDGE_CURVE('',#13688,#13687,#7401,.T.);
#16993=EDGE_CURVE('',#13688,#13686,#7402,.T.);
#16994=EDGE_CURVE('',#13686,#13689,#12851,.T.);
#16995=EDGE_CURVE('',#13689,#13688,#7403,.T.);
#16996=EDGE_CURVE('',#13689,#13690,#7404,.T.);
#16997=EDGE_CURVE('',#13687,#13690,#7405,.T.);
#16998=EDGE_CURVE('',#13690,#13685,#12852,.T.);
#16999=EDGE_CURVE('',#13691,#13692,#7406,.T.);
#17000=EDGE_CURVE('',#13691,#13693,#7407,.T.);
#17001=EDGE_CURVE('',#13694,#13693,#7408,.T.);
#17002=EDGE_CURVE('',#13694,#13692,#7409,.T.);
#17003=EDGE_CURVE('',#13692,#13695,#12853,.T.);
#17004=EDGE_CURVE('',#13695,#13694,#7410,.T.);
#17005=EDGE_CURVE('',#13695,#13696,#7411,.T.);
#17006=EDGE_CURVE('',#13693,#13696,#7412,.T.);
#17007=EDGE_CURVE('',#13696,#13691,#12854,.T.);
#17008=EDGE_CURVE('',#13697,#13698,#7413,.T.);
#17009=EDGE_CURVE('',#13697,#13699,#7414,.T.);
#17010=EDGE_CURVE('',#13700,#13699,#7415,.T.);
#17011=EDGE_CURVE('',#13700,#13698,#7416,.T.);
#17012=EDGE_CURVE('',#13698,#13701,#12855,.T.);
#17013=EDGE_CURVE('',#13701,#13700,#7417,.T.);
#17014=EDGE_CURVE('',#13701,#13702,#7418,.T.);
#17015=EDGE_CURVE('',#13699,#13702,#7419,.T.);
#17016=EDGE_CURVE('',#13702,#13697,#12856,.T.);
#17017=EDGE_CURVE('',#13703,#13704,#7420,.T.);
#17018=EDGE_CURVE('',#13703,#13705,#7421,.T.);
#17019=EDGE_CURVE('',#13706,#13705,#7422,.T.);
#17020=EDGE_CURVE('',#13706,#13704,#7423,.T.);
#17021=EDGE_CURVE('',#13704,#13707,#12857,.T.);
#17022=EDGE_CURVE('',#13707,#13706,#7424,.T.);
#17023=EDGE_CURVE('',#13707,#13708,#7425,.T.);
#17024=EDGE_CURVE('',#13705,#13708,#7426,.T.);
#17025=EDGE_CURVE('',#13708,#13703,#12858,.T.);
#17026=EDGE_CURVE('',#13709,#13710,#7427,.T.);
#17027=EDGE_CURVE('',#13709,#13711,#7428,.T.);
#17028=EDGE_CURVE('',#13712,#13711,#7429,.T.);
#17029=EDGE_CURVE('',#13712,#13710,#7430,.T.);
#17030=EDGE_CURVE('',#13710,#13713,#12859,.T.);
#17031=EDGE_CURVE('',#13713,#13712,#7431,.T.);
#17032=EDGE_CURVE('',#13713,#13714,#7432,.T.);
#17033=EDGE_CURVE('',#13711,#13714,#7433,.T.);
#17034=EDGE_CURVE('',#13714,#13709,#12860,.T.);
#17035=EDGE_CURVE('',#13715,#13716,#7434,.T.);
#17036=EDGE_CURVE('',#13715,#13717,#7435,.T.);
#17037=EDGE_CURVE('',#13718,#13717,#7436,.T.);
#17038=EDGE_CURVE('',#13718,#13716,#7437,.T.);
#17039=EDGE_CURVE('',#13716,#13719,#12861,.T.);
#17040=EDGE_CURVE('',#13719,#13718,#7438,.T.);
#17041=EDGE_CURVE('',#13719,#13720,#7439,.T.);
#17042=EDGE_CURVE('',#13717,#13720,#7440,.T.);
#17043=EDGE_CURVE('',#13720,#13715,#12862,.T.);
#17044=EDGE_CURVE('',#13721,#13722,#7441,.T.);
#17045=EDGE_CURVE('',#13721,#13723,#7442,.T.);
#17046=EDGE_CURVE('',#13724,#13723,#7443,.T.);
#17047=EDGE_CURVE('',#13724,#13722,#7444,.T.);
#17048=EDGE_CURVE('',#13722,#13725,#12863,.T.);
#17049=EDGE_CURVE('',#13726,#13724,#7445,.T.);
#17050=EDGE_CURVE('',#13725,#13726,#12864,.T.);
#17051=EDGE_CURVE('',#13726,#13727,#7446,.T.);
#17052=EDGE_CURVE('',#13723,#13727,#7447,.T.);
#17053=EDGE_CURVE('',#13727,#13728,#12865,.T.);
#17054=EDGE_CURVE('',#13728,#13721,#12866,.T.);
#17055=EDGE_CURVE('',#13729,#13730,#7448,.T.);
#17056=EDGE_CURVE('',#13729,#13731,#7449,.T.);
#17057=EDGE_CURVE('',#13732,#13731,#7450,.T.);
#17058=EDGE_CURVE('',#13732,#13730,#7451,.T.);
#17059=EDGE_CURVE('',#13730,#13733,#12867,.T.);
#17060=EDGE_CURVE('',#13733,#13732,#7452,.T.);
#17061=EDGE_CURVE('',#13733,#13734,#7453,.T.);
#17062=EDGE_CURVE('',#13731,#13734,#7454,.T.);
#17063=EDGE_CURVE('',#13734,#13729,#12868,.T.);
#17064=EDGE_CURVE('',#13735,#13736,#7455,.T.);
#17065=EDGE_CURVE('',#13735,#13737,#7456,.T.);
#17066=EDGE_CURVE('',#13738,#13737,#7457,.T.);
#17067=EDGE_CURVE('',#13738,#13736,#7458,.T.);
#17068=EDGE_CURVE('',#13736,#13739,#12869,.T.);
#17069=EDGE_CURVE('',#13739,#13738,#7459,.T.);
#17070=EDGE_CURVE('',#13739,#13740,#7460,.T.);
#17071=EDGE_CURVE('',#13737,#13740,#7461,.T.);
#17072=EDGE_CURVE('',#13740,#13735,#12870,.T.);
#17073=EDGE_CURVE('',#13741,#13742,#7462,.T.);
#17074=EDGE_CURVE('',#13741,#13743,#7463,.T.);
#17075=EDGE_CURVE('',#13744,#13743,#7464,.T.);
#17076=EDGE_CURVE('',#13744,#13742,#7465,.T.);
#17077=EDGE_CURVE('',#13742,#13745,#12871,.T.);
#17078=EDGE_CURVE('',#13745,#13744,#7466,.T.);
#17079=EDGE_CURVE('',#13745,#13746,#7467,.T.);
#17080=EDGE_CURVE('',#13743,#13746,#7468,.T.);
#17081=EDGE_CURVE('',#13746,#13741,#12872,.T.);
#17082=EDGE_CURVE('',#13747,#13748,#7469,.T.);
#17083=EDGE_CURVE('',#13747,#13749,#7470,.T.);
#17084=EDGE_CURVE('',#13750,#13749,#7471,.T.);
#17085=EDGE_CURVE('',#13750,#13748,#7472,.T.);
#17086=EDGE_CURVE('',#13748,#13751,#12873,.T.);
#17087=EDGE_CURVE('',#13751,#13750,#7473,.T.);
#17088=EDGE_CURVE('',#13751,#13752,#7474,.T.);
#17089=EDGE_CURVE('',#13749,#13752,#7475,.T.);
#17090=EDGE_CURVE('',#13752,#13747,#12874,.T.);
#17091=EDGE_CURVE('',#13753,#13754,#7476,.T.);
#17092=EDGE_CURVE('',#13753,#13755,#7477,.T.);
#17093=EDGE_CURVE('',#13756,#13755,#7478,.T.);
#17094=EDGE_CURVE('',#13756,#13754,#7479,.T.);
#17095=EDGE_CURVE('',#13754,#13757,#12875,.T.);
#17096=EDGE_CURVE('',#13757,#13756,#7480,.T.);
#17097=EDGE_CURVE('',#13757,#13758,#7481,.T.);
#17098=EDGE_CURVE('',#13755,#13758,#7482,.T.);
#17099=EDGE_CURVE('',#13758,#13753,#12876,.T.);
#17100=EDGE_CURVE('',#13759,#13760,#7483,.T.);
#17101=EDGE_CURVE('',#13759,#13761,#7484,.T.);
#17102=EDGE_CURVE('',#13762,#13761,#7485,.T.);
#17103=EDGE_CURVE('',#13762,#13760,#7486,.T.);
#17104=EDGE_CURVE('',#13760,#13763,#12877,.T.);
#17105=EDGE_CURVE('',#13763,#13762,#7487,.T.);
#17106=EDGE_CURVE('',#13763,#13764,#7488,.T.);
#17107=EDGE_CURVE('',#13761,#13764,#7489,.T.);
#17108=EDGE_CURVE('',#13764,#13759,#12878,.T.);
#17109=EDGE_CURVE('',#13765,#13766,#7490,.T.);
#17110=EDGE_CURVE('',#13765,#13767,#7491,.T.);
#17111=EDGE_CURVE('',#13768,#13767,#7492,.T.);
#17112=EDGE_CURVE('',#13768,#13766,#7493,.T.);
#17113=EDGE_CURVE('',#13766,#13769,#12879,.T.);
#17114=EDGE_CURVE('',#13769,#13768,#7494,.T.);
#17115=EDGE_CURVE('',#13769,#13770,#7495,.T.);
#17116=EDGE_CURVE('',#13767,#13770,#7496,.T.);
#17117=EDGE_CURVE('',#13770,#13765,#12880,.T.);
#17118=EDGE_CURVE('',#13771,#13772,#7497,.T.);
#17119=EDGE_CURVE('',#13771,#13773,#7498,.T.);
#17120=EDGE_CURVE('',#13774,#13773,#7499,.T.);
#17121=EDGE_CURVE('',#13774,#13772,#7500,.T.);
#17122=EDGE_CURVE('',#13772,#13775,#12881,.T.);
#17123=EDGE_CURVE('',#13775,#13774,#7501,.T.);
#17124=EDGE_CURVE('',#13775,#13776,#7502,.T.);
#17125=EDGE_CURVE('',#13773,#13776,#7503,.T.);
#17126=EDGE_CURVE('',#13776,#13771,#12882,.T.);
#17127=EDGE_CURVE('',#13777,#13778,#7504,.T.);
#17128=EDGE_CURVE('',#13777,#13779,#7505,.T.);
#17129=EDGE_CURVE('',#13780,#13779,#7506,.T.);
#17130=EDGE_CURVE('',#13780,#13778,#7507,.T.);
#17131=EDGE_CURVE('',#13778,#13781,#12883,.T.);
#17132=EDGE_CURVE('',#13781,#13780,#7508,.T.);
#17133=EDGE_CURVE('',#13781,#13782,#7509,.T.);
#17134=EDGE_CURVE('',#13779,#13782,#7510,.T.);
#17135=EDGE_CURVE('',#13782,#13777,#12884,.T.);
#17136=EDGE_CURVE('',#13783,#13784,#7511,.T.);
#17137=EDGE_CURVE('',#13783,#13785,#7512,.T.);
#17138=EDGE_CURVE('',#13786,#13785,#7513,.T.);
#17139=EDGE_CURVE('',#13786,#13784,#7514,.T.);
#17140=EDGE_CURVE('',#13784,#13787,#12885,.T.);
#17141=EDGE_CURVE('',#13787,#13786,#7515,.T.);
#17142=EDGE_CURVE('',#13787,#13788,#7516,.T.);
#17143=EDGE_CURVE('',#13785,#13788,#7517,.T.);
#17144=EDGE_CURVE('',#13788,#13783,#12886,.T.);
#17145=EDGE_CURVE('',#13789,#13790,#7518,.T.);
#17146=EDGE_CURVE('',#13789,#13791,#7519,.T.);
#17147=EDGE_CURVE('',#13792,#13791,#7520,.T.);
#17148=EDGE_CURVE('',#13792,#13790,#7521,.T.);
#17149=EDGE_CURVE('',#13790,#13793,#12887,.T.);
#17150=EDGE_CURVE('',#13793,#13792,#7522,.T.);
#17151=EDGE_CURVE('',#13793,#13794,#7523,.T.);
#17152=EDGE_CURVE('',#13791,#13794,#7524,.T.);
#17153=EDGE_CURVE('',#13794,#13789,#12888,.T.);
#17154=EDGE_CURVE('',#13795,#13796,#7525,.T.);
#17155=EDGE_CURVE('',#13795,#13797,#7526,.T.);
#17156=EDGE_CURVE('',#13798,#13797,#7527,.T.);
#17157=EDGE_CURVE('',#13798,#13796,#7528,.T.);
#17158=EDGE_CURVE('',#13796,#13799,#12889,.T.);
#17159=EDGE_CURVE('',#13799,#13798,#7529,.T.);
#17160=EDGE_CURVE('',#13799,#13800,#7530,.T.);
#17161=EDGE_CURVE('',#13797,#13800,#7531,.T.);
#17162=EDGE_CURVE('',#13800,#13795,#12890,.T.);
#17163=EDGE_CURVE('',#13801,#13802,#7532,.T.);
#17164=EDGE_CURVE('',#13801,#13803,#7533,.T.);
#17165=EDGE_CURVE('',#13804,#13803,#7534,.T.);
#17166=EDGE_CURVE('',#13804,#13802,#7535,.T.);
#17167=EDGE_CURVE('',#13802,#13805,#12891,.T.);
#17168=EDGE_CURVE('',#13805,#13804,#7536,.T.);
#17169=EDGE_CURVE('',#13805,#13806,#7537,.T.);
#17170=EDGE_CURVE('',#13803,#13806,#7538,.T.);
#17171=EDGE_CURVE('',#13806,#13801,#12892,.T.);
#17172=EDGE_CURVE('',#13807,#13808,#7539,.T.);
#17173=EDGE_CURVE('',#13807,#13809,#7540,.T.);
#17174=EDGE_CURVE('',#13810,#13809,#7541,.T.);
#17175=EDGE_CURVE('',#13810,#13808,#7542,.T.);
#17176=EDGE_CURVE('',#13808,#13811,#12893,.T.);
#17177=EDGE_CURVE('',#13811,#13810,#7543,.T.);
#17178=EDGE_CURVE('',#13811,#13812,#7544,.T.);
#17179=EDGE_CURVE('',#13809,#13812,#7545,.T.);
#17180=EDGE_CURVE('',#13812,#13807,#12894,.T.);
#17181=EDGE_CURVE('',#13813,#13814,#7546,.T.);
#17182=EDGE_CURVE('',#13813,#13815,#7547,.T.);
#17183=EDGE_CURVE('',#13816,#13815,#7548,.T.);
#17184=EDGE_CURVE('',#13816,#13814,#7549,.T.);
#17185=EDGE_CURVE('',#13814,#13817,#12895,.T.);
#17186=EDGE_CURVE('',#13817,#13816,#7550,.T.);
#17187=EDGE_CURVE('',#13817,#13818,#7551,.T.);
#17188=EDGE_CURVE('',#13815,#13818,#7552,.T.);
#17189=EDGE_CURVE('',#13818,#13813,#12896,.T.);
#17190=EDGE_CURVE('',#13819,#13820,#7553,.T.);
#17191=EDGE_CURVE('',#13819,#13821,#7554,.T.);
#17192=EDGE_CURVE('',#13822,#13821,#7555,.T.);
#17193=EDGE_CURVE('',#13822,#13820,#7556,.T.);
#17194=EDGE_CURVE('',#13820,#13823,#12897,.T.);
#17195=EDGE_CURVE('',#13823,#13822,#7557,.T.);
#17196=EDGE_CURVE('',#13823,#13824,#7558,.T.);
#17197=EDGE_CURVE('',#13821,#13824,#7559,.T.);
#17198=EDGE_CURVE('',#13824,#13819,#12898,.T.);
#17199=EDGE_CURVE('',#13825,#13826,#7560,.T.);
#17200=EDGE_CURVE('',#13825,#13827,#7561,.T.);
#17201=EDGE_CURVE('',#13828,#13827,#7562,.T.);
#17202=EDGE_CURVE('',#13828,#13826,#7563,.T.);
#17203=EDGE_CURVE('',#13826,#13829,#12899,.T.);
#17204=EDGE_CURVE('',#13829,#13828,#7564,.T.);
#17205=EDGE_CURVE('',#13829,#13830,#7565,.T.);
#17206=EDGE_CURVE('',#13827,#13830,#7566,.T.);
#17207=EDGE_CURVE('',#13830,#13825,#12900,.T.);
#17208=EDGE_CURVE('',#13831,#13832,#7567,.T.);
#17209=EDGE_CURVE('',#13831,#13833,#7568,.T.);
#17210=EDGE_CURVE('',#13834,#13833,#7569,.T.);
#17211=EDGE_CURVE('',#13834,#13832,#7570,.T.);
#17212=EDGE_CURVE('',#13832,#13835,#12901,.T.);
#17213=EDGE_CURVE('',#13835,#13834,#7571,.T.);
#17214=EDGE_CURVE('',#13835,#13836,#7572,.T.);
#17215=EDGE_CURVE('',#13833,#13836,#7573,.T.);
#17216=EDGE_CURVE('',#13836,#13831,#12902,.T.);
#17217=EDGE_CURVE('',#13837,#13593,#7574,.T.);
#17218=EDGE_CURVE('',#13837,#13838,#7575,.T.);
#17219=EDGE_CURVE('',#13594,#13838,#7576,.T.);
#17220=EDGE_CURVE('',#13600,#13598,#12903,.T.);
#17221=EDGE_CURVE('',#13838,#13839,#7577,.T.);
#17222=EDGE_CURVE('',#13595,#13839,#7578,.T.);
#17223=EDGE_CURVE('',#13839,#13837,#12904,.T.);
#17224=EDGE_CURVE('',#13611,#13607,#12905,.T.);
#17225=EDGE_CURVE('',#13610,#13612,#12906,.T.);
#17226=EDGE_CURVE('',#13840,#13840,#12907,.T.);
#17227=EDGE_CURVE('',#13840,#13841,#7579,.T.);
#17228=EDGE_CURVE('',#13841,#13841,#12908,.T.);
#17229=EDGE_CURVE('',#13842,#13842,#12909,.T.);
#17230=EDGE_CURVE('',#13843,#13843,#12910,.T.);
#17231=EDGE_CURVE('',#13843,#13842,#7580,.T.);
#17232=EDGE_CURVE('',#13844,#13844,#12911,.T.);
#17233=EDGE_CURVE('',#13844,#13725,#7581,.T.);
#17234=EDGE_CURVE('',#13728,#13843,#7582,.T.);
#17235=EDGE_CURVE('',#13844,#13845,#7583,.T.);
#17236=EDGE_CURVE('',#13845,#13845,#12912,.T.);
#17237=EDGE_CURVE('',#13846,#13846,#12913,.T.);
#17238=EDGE_CURVE('',#13847,#13847,#12914,.T.);
#17239=EDGE_CURVE('',#13847,#13846,#7584,.T.);
#17240=EDGE_CURVE('',#13848,#13848,#12915,.T.);
#17241=EDGE_CURVE('',#13840,#13848,#7585,.T.);
#21964=ORIENTED_EDGE('',*,*,#16833,.F.);
#21965=ORIENTED_EDGE('',*,*,#16834,.F.);
#21966=ORIENTED_EDGE('',*,*,#16835,.F.);
#21967=ORIENTED_EDGE('',*,*,#16836,.F.);
#21968=ORIENTED_EDGE('',*,*,#16837,.F.);
#21969=ORIENTED_EDGE('',*,*,#16838,.F.);
#21970=ORIENTED_EDGE('',*,*,#16839,.F.);
#21971=ORIENTED_EDGE('',*,*,#16840,.F.);
#21972=ORIENTED_EDGE('',*,*,#16841,.F.);
#21973=ORIENTED_EDGE('',*,*,#16842,.F.);
#21974=ORIENTED_EDGE('',*,*,#16843,.F.);
#21975=ORIENTED_EDGE('',*,*,#16844,.F.);
#21976=ORIENTED_EDGE('',*,*,#16845,.F.);
#21977=ORIENTED_EDGE('',*,*,#16846,.F.);
#21978=ORIENTED_EDGE('',*,*,#16847,.F.);
#21979=ORIENTED_EDGE('',*,*,#16848,.F.);
#21980=ORIENTED_EDGE('',*,*,#16849,.F.);
#21981=ORIENTED_EDGE('',*,*,#16850,.F.);
#21982=ORIENTED_EDGE('',*,*,#16851,.F.);
#21983=ORIENTED_EDGE('',*,*,#16852,.T.);
#21984=ORIENTED_EDGE('',*,*,#16853,.F.);
#21985=ORIENTED_EDGE('',*,*,#16854,.F.);
#21986=ORIENTED_EDGE('',*,*,#16852,.F.);
#21987=ORIENTED_EDGE('',*,*,#16834,.T.);
#21988=ORIENTED_EDGE('',*,*,#16855,.F.);
#21989=ORIENTED_EDGE('',*,*,#16856,.T.);
#21990=ORIENTED_EDGE('',*,*,#16857,.T.);
#21991=ORIENTED_EDGE('',*,*,#16835,.T.);
#21992=ORIENTED_EDGE('',*,*,#16857,.F.);
#21993=ORIENTED_EDGE('',*,*,#16858,.T.);
#21994=ORIENTED_EDGE('',*,*,#16859,.F.);
#21995=ORIENTED_EDGE('',*,*,#16841,.T.);
#21996=ORIENTED_EDGE('',*,*,#16860,.F.);
#21997=ORIENTED_EDGE('',*,*,#16861,.T.);
#21998=ORIENTED_EDGE('',*,*,#16862,.F.);
#21999=ORIENTED_EDGE('',*,*,#16843,.T.);
#22000=ORIENTED_EDGE('',*,*,#16863,.F.);
#22001=ORIENTED_EDGE('',*,*,#16864,.T.);
#22002=ORIENTED_EDGE('',*,*,#16865,.F.);
#22003=ORIENTED_EDGE('',*,*,#16840,.T.);
#22004=ORIENTED_EDGE('',*,*,#16866,.F.);
#22005=ORIENTED_EDGE('',*,*,#16867,.T.);
#22006=ORIENTED_EDGE('',*,*,#16860,.T.);
#22007=ORIENTED_EDGE('',*,*,#16844,.T.);
#22008=ORIENTED_EDGE('',*,*,#16865,.T.);
#22009=ORIENTED_EDGE('',*,*,#16868,.T.);
#22010=ORIENTED_EDGE('',*,*,#16869,.F.);
#22011=ORIENTED_EDGE('',*,*,#16837,.T.);
#22012=ORIENTED_EDGE('',*,*,#16870,.F.);
#22013=ORIENTED_EDGE('',*,*,#16871,.T.);
#22014=ORIENTED_EDGE('',*,*,#16872,.T.);
#22015=ORIENTED_EDGE('',*,*,#16847,.T.);
#22016=ORIENTED_EDGE('',*,*,#16873,.T.);
#22017=ORIENTED_EDGE('',*,*,#16874,.T.);
#22018=ORIENTED_EDGE('',*,*,#16875,.F.);
#22019=ORIENTED_EDGE('',*,*,#16838,.T.);
#22020=ORIENTED_EDGE('',*,*,#16872,.F.);
#22021=ORIENTED_EDGE('',*,*,#16876,.T.);
#22022=ORIENTED_EDGE('',*,*,#16877,.F.);
#22023=ORIENTED_EDGE('',*,*,#16846,.T.);
#22024=ORIENTED_EDGE('',*,*,#16878,.F.);
#22025=ORIENTED_EDGE('',*,*,#16879,.T.);
#22026=ORIENTED_EDGE('',*,*,#16873,.F.);
#22027=ORIENTED_EDGE('',*,*,#16880,.F.);
#22028=ORIENTED_EDGE('',*,*,#16861,.F.);
#22029=ORIENTED_EDGE('',*,*,#16867,.F.);
#22030=ORIENTED_EDGE('',*,*,#16881,.F.);
#22031=ORIENTED_EDGE('',*,*,#16868,.F.);
#22032=ORIENTED_EDGE('',*,*,#16864,.F.);
#22033=ORIENTED_EDGE('',*,*,#16882,.F.);
#22034=ORIENTED_EDGE('',*,*,#16883,.T.);
#22035=ORIENTED_EDGE('',*,*,#16884,.F.);
#22036=ORIENTED_EDGE('',*,*,#16885,.T.);
#22037=ORIENTED_EDGE('',*,*,#16886,.F.);
#22038=ORIENTED_EDGE('',*,*,#16885,.F.);
#22039=ORIENTED_EDGE('',*,*,#16887,.F.);
#22040=ORIENTED_EDGE('',*,*,#16888,.F.);
#22041=ORIENTED_EDGE('',*,*,#16887,.T.);
#22042=ORIENTED_EDGE('',*,*,#16884,.T.);
#22043=ORIENTED_EDGE('',*,*,#16889,.T.);
#22044=ORIENTED_EDGE('',*,*,#16890,.F.);
#22045=ORIENTED_EDGE('',*,*,#16889,.F.);
#22046=ORIENTED_EDGE('',*,*,#16883,.F.);
#22047=ORIENTED_EDGE('',*,*,#16891,.F.);
#22048=ORIENTED_EDGE('',*,*,#16892,.T.);
#22049=ORIENTED_EDGE('',*,*,#16893,.F.);
#22050=ORIENTED_EDGE('',*,*,#16894,.T.);
#22051=ORIENTED_EDGE('',*,*,#16895,.F.);
#22052=ORIENTED_EDGE('',*,*,#16894,.F.);
#22053=ORIENTED_EDGE('',*,*,#16896,.F.);
#22054=ORIENTED_EDGE('',*,*,#16897,.F.);
#22055=ORIENTED_EDGE('',*,*,#16896,.T.);
#22056=ORIENTED_EDGE('',*,*,#16893,.T.);
#22057=ORIENTED_EDGE('',*,*,#16898,.T.);
#22058=ORIENTED_EDGE('',*,*,#16899,.F.);
#22059=ORIENTED_EDGE('',*,*,#16898,.F.);
#22060=ORIENTED_EDGE('',*,*,#16892,.F.);
#22061=ORIENTED_EDGE('',*,*,#16900,.F.);
#22062=ORIENTED_EDGE('',*,*,#16901,.T.);
#22063=ORIENTED_EDGE('',*,*,#16902,.F.);
#22064=ORIENTED_EDGE('',*,*,#16903,.T.);
#22065=ORIENTED_EDGE('',*,*,#16904,.F.);
#22066=ORIENTED_EDGE('',*,*,#16903,.F.);
#22067=ORIENTED_EDGE('',*,*,#16905,.F.);
#22068=ORIENTED_EDGE('',*,*,#16906,.F.);
#22069=ORIENTED_EDGE('',*,*,#16905,.T.);
#22070=ORIENTED_EDGE('',*,*,#16902,.T.);
#22071=ORIENTED_EDGE('',*,*,#16907,.T.);
#22072=ORIENTED_EDGE('',*,*,#16908,.F.);
#22073=ORIENTED_EDGE('',*,*,#16907,.F.);
#22074=ORIENTED_EDGE('',*,*,#16901,.F.);
#22075=ORIENTED_EDGE('',*,*,#16909,.F.);
#22076=ORIENTED_EDGE('',*,*,#16910,.T.);
#22077=ORIENTED_EDGE('',*,*,#16911,.F.);
#22078=ORIENTED_EDGE('',*,*,#16912,.T.);
#22079=ORIENTED_EDGE('',*,*,#16913,.F.);
#22080=ORIENTED_EDGE('',*,*,#16912,.F.);
#22081=ORIENTED_EDGE('',*,*,#16914,.F.);
#22082=ORIENTED_EDGE('',*,*,#16915,.F.);
#22083=ORIENTED_EDGE('',*,*,#16914,.T.);
#22084=ORIENTED_EDGE('',*,*,#16911,.T.);
#22085=ORIENTED_EDGE('',*,*,#16916,.T.);
#22086=ORIENTED_EDGE('',*,*,#16917,.F.);
#22087=ORIENTED_EDGE('',*,*,#16916,.F.);
#22088=ORIENTED_EDGE('',*,*,#16910,.F.);
#22089=ORIENTED_EDGE('',*,*,#16918,.F.);
#22090=ORIENTED_EDGE('',*,*,#16919,.T.);
#22091=ORIENTED_EDGE('',*,*,#16920,.F.);
#22092=ORIENTED_EDGE('',*,*,#16921,.T.);
#22093=ORIENTED_EDGE('',*,*,#16922,.F.);
#22094=ORIENTED_EDGE('',*,*,#16921,.F.);
#22095=ORIENTED_EDGE('',*,*,#16923,.F.);
#22096=ORIENTED_EDGE('',*,*,#16924,.F.);
#22097=ORIENTED_EDGE('',*,*,#16923,.T.);
#22098=ORIENTED_EDGE('',*,*,#16920,.T.);
#22099=ORIENTED_EDGE('',*,*,#16925,.T.);
#22100=ORIENTED_EDGE('',*,*,#16926,.F.);
#22101=ORIENTED_EDGE('',*,*,#16925,.F.);
#22102=ORIENTED_EDGE('',*,*,#16919,.F.);
#22103=ORIENTED_EDGE('',*,*,#16927,.F.);
#22104=ORIENTED_EDGE('',*,*,#16928,.T.);
#22105=ORIENTED_EDGE('',*,*,#16929,.F.);
#22106=ORIENTED_EDGE('',*,*,#16930,.T.);
#22107=ORIENTED_EDGE('',*,*,#16931,.F.);
#22108=ORIENTED_EDGE('',*,*,#16930,.F.);
#22109=ORIENTED_EDGE('',*,*,#16932,.F.);
#22110=ORIENTED_EDGE('',*,*,#16933,.F.);
#22111=ORIENTED_EDGE('',*,*,#16932,.T.);
#22112=ORIENTED_EDGE('',*,*,#16929,.T.);
#22113=ORIENTED_EDGE('',*,*,#16934,.T.);
#22114=ORIENTED_EDGE('',*,*,#16935,.F.);
#22115=ORIENTED_EDGE('',*,*,#16934,.F.);
#22116=ORIENTED_EDGE('',*,*,#16928,.F.);
#22117=ORIENTED_EDGE('',*,*,#16936,.F.);
#22118=ORIENTED_EDGE('',*,*,#16937,.T.);
#22119=ORIENTED_EDGE('',*,*,#16938,.F.);
#22120=ORIENTED_EDGE('',*,*,#16939,.T.);
#22121=ORIENTED_EDGE('',*,*,#16940,.F.);
#22122=ORIENTED_EDGE('',*,*,#16939,.F.);
#22123=ORIENTED_EDGE('',*,*,#16941,.F.);
#22124=ORIENTED_EDGE('',*,*,#16942,.F.);
#22125=ORIENTED_EDGE('',*,*,#16941,.T.);
#22126=ORIENTED_EDGE('',*,*,#16938,.T.);
#22127=ORIENTED_EDGE('',*,*,#16943,.T.);
#22128=ORIENTED_EDGE('',*,*,#16944,.F.);
#22129=ORIENTED_EDGE('',*,*,#16943,.F.);
#22130=ORIENTED_EDGE('',*,*,#16937,.F.);
#22131=ORIENTED_EDGE('',*,*,#16945,.F.);
#22132=ORIENTED_EDGE('',*,*,#16946,.T.);
#22133=ORIENTED_EDGE('',*,*,#16947,.F.);
#22134=ORIENTED_EDGE('',*,*,#16948,.T.);
#22135=ORIENTED_EDGE('',*,*,#16949,.F.);
#22136=ORIENTED_EDGE('',*,*,#16948,.F.);
#22137=ORIENTED_EDGE('',*,*,#16950,.F.);
#22138=ORIENTED_EDGE('',*,*,#16951,.F.);
#22139=ORIENTED_EDGE('',*,*,#16950,.T.);
#22140=ORIENTED_EDGE('',*,*,#16947,.T.);
#22141=ORIENTED_EDGE('',*,*,#16952,.T.);
#22142=ORIENTED_EDGE('',*,*,#16953,.F.);
#22143=ORIENTED_EDGE('',*,*,#16952,.F.);
#22144=ORIENTED_EDGE('',*,*,#16946,.F.);
#22145=ORIENTED_EDGE('',*,*,#16954,.F.);
#22146=ORIENTED_EDGE('',*,*,#16955,.T.);
#22147=ORIENTED_EDGE('',*,*,#16956,.F.);
#22148=ORIENTED_EDGE('',*,*,#16957,.T.);
#22149=ORIENTED_EDGE('',*,*,#16958,.F.);
#22150=ORIENTED_EDGE('',*,*,#16957,.F.);
#22151=ORIENTED_EDGE('',*,*,#16959,.F.);
#22152=ORIENTED_EDGE('',*,*,#16960,.F.);
#22153=ORIENTED_EDGE('',*,*,#16959,.T.);
#22154=ORIENTED_EDGE('',*,*,#16956,.T.);
#22155=ORIENTED_EDGE('',*,*,#16961,.T.);
#22156=ORIENTED_EDGE('',*,*,#16962,.F.);
#22157=ORIENTED_EDGE('',*,*,#16961,.F.);
#22158=ORIENTED_EDGE('',*,*,#16955,.F.);
#22159=ORIENTED_EDGE('',*,*,#16963,.F.);
#22160=ORIENTED_EDGE('',*,*,#16964,.T.);
#22161=ORIENTED_EDGE('',*,*,#16965,.F.);
#22162=ORIENTED_EDGE('',*,*,#16966,.T.);
#22163=ORIENTED_EDGE('',*,*,#16967,.F.);
#22164=ORIENTED_EDGE('',*,*,#16966,.F.);
#22165=ORIENTED_EDGE('',*,*,#16968,.F.);
#22166=ORIENTED_EDGE('',*,*,#16969,.F.);
#22167=ORIENTED_EDGE('',*,*,#16968,.T.);
#22168=ORIENTED_EDGE('',*,*,#16965,.T.);
#22169=ORIENTED_EDGE('',*,*,#16970,.T.);
#22170=ORIENTED_EDGE('',*,*,#16971,.F.);
#22171=ORIENTED_EDGE('',*,*,#16970,.F.);
#22172=ORIENTED_EDGE('',*,*,#16964,.F.);
#22173=ORIENTED_EDGE('',*,*,#16972,.F.);
#22174=ORIENTED_EDGE('',*,*,#16973,.T.);
#22175=ORIENTED_EDGE('',*,*,#16974,.F.);
#22176=ORIENTED_EDGE('',*,*,#16975,.T.);
#22177=ORIENTED_EDGE('',*,*,#16976,.F.);
#22178=ORIENTED_EDGE('',*,*,#16975,.F.);
#22179=ORIENTED_EDGE('',*,*,#16977,.F.);
#22180=ORIENTED_EDGE('',*,*,#16978,.F.);
#22181=ORIENTED_EDGE('',*,*,#16977,.T.);
#22182=ORIENTED_EDGE('',*,*,#16974,.T.);
#22183=ORIENTED_EDGE('',*,*,#16979,.T.);
#22184=ORIENTED_EDGE('',*,*,#16980,.F.);
#22185=ORIENTED_EDGE('',*,*,#16979,.F.);
#22186=ORIENTED_EDGE('',*,*,#16973,.F.);
#22187=ORIENTED_EDGE('',*,*,#16981,.F.);
#22188=ORIENTED_EDGE('',*,*,#16982,.T.);
#22189=ORIENTED_EDGE('',*,*,#16983,.F.);
#22190=ORIENTED_EDGE('',*,*,#16984,.T.);
#22191=ORIENTED_EDGE('',*,*,#16985,.F.);
#22192=ORIENTED_EDGE('',*,*,#16984,.F.);
#22193=ORIENTED_EDGE('',*,*,#16986,.F.);
#22194=ORIENTED_EDGE('',*,*,#16987,.F.);
#22195=ORIENTED_EDGE('',*,*,#16986,.T.);
#22196=ORIENTED_EDGE('',*,*,#16983,.T.);
#22197=ORIENTED_EDGE('',*,*,#16988,.T.);
#22198=ORIENTED_EDGE('',*,*,#16989,.F.);
#22199=ORIENTED_EDGE('',*,*,#16988,.F.);
#22200=ORIENTED_EDGE('',*,*,#16982,.F.);
#22201=ORIENTED_EDGE('',*,*,#16990,.F.);
#22202=ORIENTED_EDGE('',*,*,#16991,.T.);
#22203=ORIENTED_EDGE('',*,*,#16992,.F.);
#22204=ORIENTED_EDGE('',*,*,#16993,.T.);
#22205=ORIENTED_EDGE('',*,*,#16994,.F.);
#22206=ORIENTED_EDGE('',*,*,#16993,.F.);
#22207=ORIENTED_EDGE('',*,*,#16995,.F.);
#22208=ORIENTED_EDGE('',*,*,#16996,.F.);
#22209=ORIENTED_EDGE('',*,*,#16995,.T.);
#22210=ORIENTED_EDGE('',*,*,#16992,.T.);
#22211=ORIENTED_EDGE('',*,*,#16997,.T.);
#22212=ORIENTED_EDGE('',*,*,#16998,.F.);
#22213=ORIENTED_EDGE('',*,*,#16997,.F.);
#22214=ORIENTED_EDGE('',*,*,#16991,.F.);
#22215=ORIENTED_EDGE('',*,*,#16999,.F.);
#22216=ORIENTED_EDGE('',*,*,#17000,.T.);
#22217=ORIENTED_EDGE('',*,*,#17001,.F.);
#22218=ORIENTED_EDGE('',*,*,#17002,.T.);
#22219=ORIENTED_EDGE('',*,*,#17003,.F.);
#22220=ORIENTED_EDGE('',*,*,#17002,.F.);
#22221=ORIENTED_EDGE('',*,*,#17004,.F.);
#22222=ORIENTED_EDGE('',*,*,#17005,.F.);
#22223=ORIENTED_EDGE('',*,*,#17004,.T.);
#22224=ORIENTED_EDGE('',*,*,#17001,.T.);
#22225=ORIENTED_EDGE('',*,*,#17006,.T.);
#22226=ORIENTED_EDGE('',*,*,#17007,.F.);
#22227=ORIENTED_EDGE('',*,*,#17006,.F.);
#22228=ORIENTED_EDGE('',*,*,#17000,.F.);
#22229=ORIENTED_EDGE('',*,*,#17008,.F.);
#22230=ORIENTED_EDGE('',*,*,#17009,.T.);
#22231=ORIENTED_EDGE('',*,*,#17010,.F.);
#22232=ORIENTED_EDGE('',*,*,#17011,.T.);
#22233=ORIENTED_EDGE('',*,*,#17012,.F.);
#22234=ORIENTED_EDGE('',*,*,#17011,.F.);
#22235=ORIENTED_EDGE('',*,*,#17013,.F.);
#22236=ORIENTED_EDGE('',*,*,#17014,.F.);
#22237=ORIENTED_EDGE('',*,*,#17013,.T.);
#22238=ORIENTED_EDGE('',*,*,#17010,.T.);
#22239=ORIENTED_EDGE('',*,*,#17015,.T.);
#22240=ORIENTED_EDGE('',*,*,#17016,.F.);
#22241=ORIENTED_EDGE('',*,*,#17015,.F.);
#22242=ORIENTED_EDGE('',*,*,#17009,.F.);
#22243=ORIENTED_EDGE('',*,*,#17017,.F.);
#22244=ORIENTED_EDGE('',*,*,#17018,.T.);
#22245=ORIENTED_EDGE('',*,*,#17019,.F.);
#22246=ORIENTED_EDGE('',*,*,#17020,.T.);
#22247=ORIENTED_EDGE('',*,*,#17021,.F.);
#22248=ORIENTED_EDGE('',*,*,#17020,.F.);
#22249=ORIENTED_EDGE('',*,*,#17022,.F.);
#22250=ORIENTED_EDGE('',*,*,#17023,.F.);
#22251=ORIENTED_EDGE('',*,*,#17022,.T.);
#22252=ORIENTED_EDGE('',*,*,#17019,.T.);
#22253=ORIENTED_EDGE('',*,*,#17024,.T.);
#22254=ORIENTED_EDGE('',*,*,#17025,.F.);
#22255=ORIENTED_EDGE('',*,*,#17024,.F.);
#22256=ORIENTED_EDGE('',*,*,#17018,.F.);
#22257=ORIENTED_EDGE('',*,*,#17026,.F.);
#22258=ORIENTED_EDGE('',*,*,#17027,.T.);
#22259=ORIENTED_EDGE('',*,*,#17028,.F.);
#22260=ORIENTED_EDGE('',*,*,#17029,.T.);
#22261=ORIENTED_EDGE('',*,*,#17030,.F.);
#22262=ORIENTED_EDGE('',*,*,#17029,.F.);
#22263=ORIENTED_EDGE('',*,*,#17031,.F.);
#22264=ORIENTED_EDGE('',*,*,#17032,.F.);
#22265=ORIENTED_EDGE('',*,*,#17031,.T.);
#22266=ORIENTED_EDGE('',*,*,#17028,.T.);
#22267=ORIENTED_EDGE('',*,*,#17033,.T.);
#22268=ORIENTED_EDGE('',*,*,#17034,.F.);
#22269=ORIENTED_EDGE('',*,*,#17033,.F.);
#22270=ORIENTED_EDGE('',*,*,#17027,.F.);
#22271=ORIENTED_EDGE('',*,*,#17035,.F.);
#22272=ORIENTED_EDGE('',*,*,#17036,.T.);
#22273=ORIENTED_EDGE('',*,*,#17037,.F.);
#22274=ORIENTED_EDGE('',*,*,#17038,.T.);
#22275=ORIENTED_EDGE('',*,*,#17039,.F.);
#22276=ORIENTED_EDGE('',*,*,#17038,.F.);
#22277=ORIENTED_EDGE('',*,*,#17040,.F.);
#22278=ORIENTED_EDGE('',*,*,#17041,.F.);
#22279=ORIENTED_EDGE('',*,*,#17040,.T.);
#22280=ORIENTED_EDGE('',*,*,#17037,.T.);
#22281=ORIENTED_EDGE('',*,*,#17042,.T.);
#22282=ORIENTED_EDGE('',*,*,#17043,.F.);
#22283=ORIENTED_EDGE('',*,*,#17042,.F.);
#22284=ORIENTED_EDGE('',*,*,#17036,.F.);
#22285=ORIENTED_EDGE('',*,*,#17044,.F.);
#22286=ORIENTED_EDGE('',*,*,#17045,.T.);
#22287=ORIENTED_EDGE('',*,*,#17046,.F.);
#22288=ORIENTED_EDGE('',*,*,#17047,.T.);
#22289=ORIENTED_EDGE('',*,*,#17048,.F.);
#22290=ORIENTED_EDGE('',*,*,#17047,.F.);
#22291=ORIENTED_EDGE('',*,*,#17049,.F.);
#22292=ORIENTED_EDGE('',*,*,#17050,.F.);
#22293=ORIENTED_EDGE('',*,*,#17051,.F.);
#22294=ORIENTED_EDGE('',*,*,#17049,.T.);
#22295=ORIENTED_EDGE('',*,*,#17046,.T.);
#22296=ORIENTED_EDGE('',*,*,#17052,.T.);
#22297=ORIENTED_EDGE('',*,*,#17053,.F.);
#22298=ORIENTED_EDGE('',*,*,#17052,.F.);
#22299=ORIENTED_EDGE('',*,*,#17045,.F.);
#22300=ORIENTED_EDGE('',*,*,#17054,.F.);
#22301=ORIENTED_EDGE('',*,*,#17055,.F.);
#22302=ORIENTED_EDGE('',*,*,#17056,.T.);
#22303=ORIENTED_EDGE('',*,*,#17057,.F.);
#22304=ORIENTED_EDGE('',*,*,#17058,.T.);
#22305=ORIENTED_EDGE('',*,*,#17059,.F.);
#22306=ORIENTED_EDGE('',*,*,#17058,.F.);
#22307=ORIENTED_EDGE('',*,*,#17060,.F.);
#22308=ORIENTED_EDGE('',*,*,#17061,.F.);
#22309=ORIENTED_EDGE('',*,*,#17060,.T.);
#22310=ORIENTED_EDGE('',*,*,#17057,.T.);
#22311=ORIENTED_EDGE('',*,*,#17062,.T.);
#22312=ORIENTED_EDGE('',*,*,#17063,.F.);
#22313=ORIENTED_EDGE('',*,*,#17062,.F.);
#22314=ORIENTED_EDGE('',*,*,#17056,.F.);
#22315=ORIENTED_EDGE('',*,*,#17064,.F.);
#22316=ORIENTED_EDGE('',*,*,#17065,.T.);
#22317=ORIENTED_EDGE('',*,*,#17066,.F.);
#22318=ORIENTED_EDGE('',*,*,#17067,.T.);
#22319=ORIENTED_EDGE('',*,*,#17068,.F.);
#22320=ORIENTED_EDGE('',*,*,#17067,.F.);
#22321=ORIENTED_EDGE('',*,*,#17069,.F.);
#22322=ORIENTED_EDGE('',*,*,#17070,.F.);
#22323=ORIENTED_EDGE('',*,*,#17069,.T.);
#22324=ORIENTED_EDGE('',*,*,#17066,.T.);
#22325=ORIENTED_EDGE('',*,*,#17071,.T.);
#22326=ORIENTED_EDGE('',*,*,#17072,.F.);
#22327=ORIENTED_EDGE('',*,*,#17071,.F.);
#22328=ORIENTED_EDGE('',*,*,#17065,.F.);
#22329=ORIENTED_EDGE('',*,*,#17073,.F.);
#22330=ORIENTED_EDGE('',*,*,#17074,.T.);
#22331=ORIENTED_EDGE('',*,*,#17075,.F.);
#22332=ORIENTED_EDGE('',*,*,#17076,.T.);
#22333=ORIENTED_EDGE('',*,*,#17077,.F.);
#22334=ORIENTED_EDGE('',*,*,#17076,.F.);
#22335=ORIENTED_EDGE('',*,*,#17078,.F.);
#22336=ORIENTED_EDGE('',*,*,#17079,.F.);
#22337=ORIENTED_EDGE('',*,*,#17078,.T.);
#22338=ORIENTED_EDGE('',*,*,#17075,.T.);
#22339=ORIENTED_EDGE('',*,*,#17080,.T.);
#22340=ORIENTED_EDGE('',*,*,#17081,.F.);
#22341=ORIENTED_EDGE('',*,*,#17080,.F.);
#22342=ORIENTED_EDGE('',*,*,#17074,.F.);
#22343=ORIENTED_EDGE('',*,*,#17082,.F.);
#22344=ORIENTED_EDGE('',*,*,#17083,.T.);
#22345=ORIENTED_EDGE('',*,*,#17084,.F.);
#22346=ORIENTED_EDGE('',*,*,#17085,.T.);
#22347=ORIENTED_EDGE('',*,*,#17086,.F.);
#22348=ORIENTED_EDGE('',*,*,#17085,.F.);
#22349=ORIENTED_EDGE('',*,*,#17087,.F.);
#22350=ORIENTED_EDGE('',*,*,#17088,.F.);
#22351=ORIENTED_EDGE('',*,*,#17087,.T.);
#22352=ORIENTED_EDGE('',*,*,#17084,.T.);
#22353=ORIENTED_EDGE('',*,*,#17089,.T.);
#22354=ORIENTED_EDGE('',*,*,#17090,.F.);
#22355=ORIENTED_EDGE('',*,*,#17089,.F.);
#22356=ORIENTED_EDGE('',*,*,#17083,.F.);
#22357=ORIENTED_EDGE('',*,*,#17091,.F.);
#22358=ORIENTED_EDGE('',*,*,#17092,.T.);
#22359=ORIENTED_EDGE('',*,*,#17093,.F.);
#22360=ORIENTED_EDGE('',*,*,#17094,.T.);
#22361=ORIENTED_EDGE('',*,*,#17095,.F.);
#22362=ORIENTED_EDGE('',*,*,#17094,.F.);
#22363=ORIENTED_EDGE('',*,*,#17096,.F.);
#22364=ORIENTED_EDGE('',*,*,#17097,.F.);
#22365=ORIENTED_EDGE('',*,*,#17096,.T.);
#22366=ORIENTED_EDGE('',*,*,#17093,.T.);
#22367=ORIENTED_EDGE('',*,*,#17098,.T.);
#22368=ORIENTED_EDGE('',*,*,#17099,.F.);
#22369=ORIENTED_EDGE('',*,*,#17098,.F.);
#22370=ORIENTED_EDGE('',*,*,#17092,.F.);
#22371=ORIENTED_EDGE('',*,*,#17100,.F.);
#22372=ORIENTED_EDGE('',*,*,#17101,.T.);
#22373=ORIENTED_EDGE('',*,*,#17102,.F.);
#22374=ORIENTED_EDGE('',*,*,#17103,.T.);
#22375=ORIENTED_EDGE('',*,*,#17104,.F.);
#22376=ORIENTED_EDGE('',*,*,#17103,.F.);
#22377=ORIENTED_EDGE('',*,*,#17105,.F.);
#22378=ORIENTED_EDGE('',*,*,#17106,.F.);
#22379=ORIENTED_EDGE('',*,*,#17105,.T.);
#22380=ORIENTED_EDGE('',*,*,#17102,.T.);
#22381=ORIENTED_EDGE('',*,*,#17107,.T.);
#22382=ORIENTED_EDGE('',*,*,#17108,.F.);
#22383=ORIENTED_EDGE('',*,*,#17107,.F.);
#22384=ORIENTED_EDGE('',*,*,#17101,.F.);
#22385=ORIENTED_EDGE('',*,*,#17109,.F.);
#22386=ORIENTED_EDGE('',*,*,#17110,.T.);
#22387=ORIENTED_EDGE('',*,*,#17111,.F.);
#22388=ORIENTED_EDGE('',*,*,#17112,.T.);
#22389=ORIENTED_EDGE('',*,*,#17113,.F.);
#22390=ORIENTED_EDGE('',*,*,#17112,.F.);
#22391=ORIENTED_EDGE('',*,*,#17114,.F.);
#22392=ORIENTED_EDGE('',*,*,#17115,.F.);
#22393=ORIENTED_EDGE('',*,*,#17114,.T.);
#22394=ORIENTED_EDGE('',*,*,#17111,.T.);
#22395=ORIENTED_EDGE('',*,*,#17116,.T.);
#22396=ORIENTED_EDGE('',*,*,#17117,.F.);
#22397=ORIENTED_EDGE('',*,*,#17116,.F.);
#22398=ORIENTED_EDGE('',*,*,#17110,.F.);
#22399=ORIENTED_EDGE('',*,*,#17118,.F.);
#22400=ORIENTED_EDGE('',*,*,#17119,.T.);
#22401=ORIENTED_EDGE('',*,*,#17120,.F.);
#22402=ORIENTED_EDGE('',*,*,#17121,.T.);
#22403=ORIENTED_EDGE('',*,*,#17122,.F.);
#22404=ORIENTED_EDGE('',*,*,#17121,.F.);
#22405=ORIENTED_EDGE('',*,*,#17123,.F.);
#22406=ORIENTED_EDGE('',*,*,#17124,.F.);
#22407=ORIENTED_EDGE('',*,*,#17123,.T.);
#22408=ORIENTED_EDGE('',*,*,#17120,.T.);
#22409=ORIENTED_EDGE('',*,*,#17125,.T.);
#22410=ORIENTED_EDGE('',*,*,#17126,.F.);
#22411=ORIENTED_EDGE('',*,*,#17125,.F.);
#22412=ORIENTED_EDGE('',*,*,#17119,.F.);
#22413=ORIENTED_EDGE('',*,*,#17127,.F.);
#22414=ORIENTED_EDGE('',*,*,#17128,.T.);
#22415=ORIENTED_EDGE('',*,*,#17129,.F.);
#22416=ORIENTED_EDGE('',*,*,#17130,.T.);
#22417=ORIENTED_EDGE('',*,*,#17131,.F.);
#22418=ORIENTED_EDGE('',*,*,#17130,.F.);
#22419=ORIENTED_EDGE('',*,*,#17132,.F.);
#22420=ORIENTED_EDGE('',*,*,#17133,.F.);
#22421=ORIENTED_EDGE('',*,*,#17132,.T.);
#22422=ORIENTED_EDGE('',*,*,#17129,.T.);
#22423=ORIENTED_EDGE('',*,*,#17134,.T.);
#22424=ORIENTED_EDGE('',*,*,#17135,.F.);
#22425=ORIENTED_EDGE('',*,*,#17134,.F.);
#22426=ORIENTED_EDGE('',*,*,#17128,.F.);
#22427=ORIENTED_EDGE('',*,*,#17136,.F.);
#22428=ORIENTED_EDGE('',*,*,#17137,.T.);
#22429=ORIENTED_EDGE('',*,*,#17138,.F.);
#22430=ORIENTED_EDGE('',*,*,#17139,.T.);
#22431=ORIENTED_EDGE('',*,*,#17140,.F.);
#22432=ORIENTED_EDGE('',*,*,#17139,.F.);
#22433=ORIENTED_EDGE('',*,*,#17141,.F.);
#22434=ORIENTED_EDGE('',*,*,#17142,.F.);
#22435=ORIENTED_EDGE('',*,*,#17141,.T.);
#22436=ORIENTED_EDGE('',*,*,#17138,.T.);
#22437=ORIENTED_EDGE('',*,*,#17143,.T.);
#22438=ORIENTED_EDGE('',*,*,#17144,.F.);
#22439=ORIENTED_EDGE('',*,*,#17143,.F.);
#22440=ORIENTED_EDGE('',*,*,#17137,.F.);
#22441=ORIENTED_EDGE('',*,*,#17145,.F.);
#22442=ORIENTED_EDGE('',*,*,#17146,.T.);
#22443=ORIENTED_EDGE('',*,*,#17147,.F.);
#22444=ORIENTED_EDGE('',*,*,#17148,.T.);
#22445=ORIENTED_EDGE('',*,*,#17149,.F.);
#22446=ORIENTED_EDGE('',*,*,#17148,.F.);
#22447=ORIENTED_EDGE('',*,*,#17150,.F.);
#22448=ORIENTED_EDGE('',*,*,#17151,.F.);
#22449=ORIENTED_EDGE('',*,*,#17150,.T.);
#22450=ORIENTED_EDGE('',*,*,#17147,.T.);
#22451=ORIENTED_EDGE('',*,*,#17152,.T.);
#22452=ORIENTED_EDGE('',*,*,#17153,.F.);
#22453=ORIENTED_EDGE('',*,*,#17152,.F.);
#22454=ORIENTED_EDGE('',*,*,#17146,.F.);
#22455=ORIENTED_EDGE('',*,*,#17154,.F.);
#22456=ORIENTED_EDGE('',*,*,#17155,.T.);
#22457=ORIENTED_EDGE('',*,*,#17156,.F.);
#22458=ORIENTED_EDGE('',*,*,#17157,.T.);
#22459=ORIENTED_EDGE('',*,*,#17158,.F.);
#22460=ORIENTED_EDGE('',*,*,#17157,.F.);
#22461=ORIENTED_EDGE('',*,*,#17159,.F.);
#22462=ORIENTED_EDGE('',*,*,#17160,.F.);
#22463=ORIENTED_EDGE('',*,*,#17159,.T.);
#22464=ORIENTED_EDGE('',*,*,#17156,.T.);
#22465=ORIENTED_EDGE('',*,*,#17161,.T.);
#22466=ORIENTED_EDGE('',*,*,#17162,.F.);
#22467=ORIENTED_EDGE('',*,*,#17161,.F.);
#22468=ORIENTED_EDGE('',*,*,#17155,.F.);
#22469=ORIENTED_EDGE('',*,*,#17163,.F.);
#22470=ORIENTED_EDGE('',*,*,#17164,.T.);
#22471=ORIENTED_EDGE('',*,*,#17165,.F.);
#22472=ORIENTED_EDGE('',*,*,#17166,.T.);
#22473=ORIENTED_EDGE('',*,*,#17167,.F.);
#22474=ORIENTED_EDGE('',*,*,#17166,.F.);
#22475=ORIENTED_EDGE('',*,*,#17168,.F.);
#22476=ORIENTED_EDGE('',*,*,#17169,.F.);
#22477=ORIENTED_EDGE('',*,*,#17168,.T.);
#22478=ORIENTED_EDGE('',*,*,#17165,.T.);
#22479=ORIENTED_EDGE('',*,*,#17170,.T.);
#22480=ORIENTED_EDGE('',*,*,#17171,.F.);
#22481=ORIENTED_EDGE('',*,*,#17170,.F.);
#22482=ORIENTED_EDGE('',*,*,#17164,.F.);
#22483=ORIENTED_EDGE('',*,*,#17172,.F.);
#22484=ORIENTED_EDGE('',*,*,#17173,.T.);
#22485=ORIENTED_EDGE('',*,*,#17174,.F.);
#22486=ORIENTED_EDGE('',*,*,#17175,.T.);
#22487=ORIENTED_EDGE('',*,*,#17176,.F.);
#22488=ORIENTED_EDGE('',*,*,#17175,.F.);
#22489=ORIENTED_EDGE('',*,*,#17177,.F.);
#22490=ORIENTED_EDGE('',*,*,#17178,.F.);
#22491=ORIENTED_EDGE('',*,*,#17177,.T.);
#22492=ORIENTED_EDGE('',*,*,#17174,.T.);
#22493=ORIENTED_EDGE('',*,*,#17179,.T.);
#22494=ORIENTED_EDGE('',*,*,#17180,.F.);
#22495=ORIENTED_EDGE('',*,*,#17179,.F.);
#22496=ORIENTED_EDGE('',*,*,#17173,.F.);
#22497=ORIENTED_EDGE('',*,*,#17181,.F.);
#22498=ORIENTED_EDGE('',*,*,#17182,.T.);
#22499=ORIENTED_EDGE('',*,*,#17183,.F.);
#22500=ORIENTED_EDGE('',*,*,#17184,.T.);
#22501=ORIENTED_EDGE('',*,*,#17185,.F.);
#22502=ORIENTED_EDGE('',*,*,#17184,.F.);
#22503=ORIENTED_EDGE('',*,*,#17186,.F.);
#22504=ORIENTED_EDGE('',*,*,#17187,.F.);
#22505=ORIENTED_EDGE('',*,*,#17186,.T.);
#22506=ORIENTED_EDGE('',*,*,#17183,.T.);
#22507=ORIENTED_EDGE('',*,*,#17188,.T.);
#22508=ORIENTED_EDGE('',*,*,#17189,.F.);
#22509=ORIENTED_EDGE('',*,*,#17188,.F.);
#22510=ORIENTED_EDGE('',*,*,#17182,.F.);
#22511=ORIENTED_EDGE('',*,*,#17190,.F.);
#22512=ORIENTED_EDGE('',*,*,#17191,.T.);
#22513=ORIENTED_EDGE('',*,*,#17192,.F.);
#22514=ORIENTED_EDGE('',*,*,#17193,.T.);
#22515=ORIENTED_EDGE('',*,*,#17194,.F.);
#22516=ORIENTED_EDGE('',*,*,#17193,.F.);
#22517=ORIENTED_EDGE('',*,*,#17195,.F.);
#22518=ORIENTED_EDGE('',*,*,#17196,.F.);
#22519=ORIENTED_EDGE('',*,*,#17195,.T.);
#22520=ORIENTED_EDGE('',*,*,#17192,.T.);
#22521=ORIENTED_EDGE('',*,*,#17197,.T.);
#22522=ORIENTED_EDGE('',*,*,#17198,.F.);
#22523=ORIENTED_EDGE('',*,*,#17197,.F.);
#22524=ORIENTED_EDGE('',*,*,#17191,.F.);
#22525=ORIENTED_EDGE('',*,*,#17199,.F.);
#22526=ORIENTED_EDGE('',*,*,#17200,.T.);
#22527=ORIENTED_EDGE('',*,*,#17201,.F.);
#22528=ORIENTED_EDGE('',*,*,#17202,.T.);
#22529=ORIENTED_EDGE('',*,*,#17203,.F.);
#22530=ORIENTED_EDGE('',*,*,#17202,.F.);
#22531=ORIENTED_EDGE('',*,*,#17204,.F.);
#22532=ORIENTED_EDGE('',*,*,#17205,.F.);
#22533=ORIENTED_EDGE('',*,*,#17204,.T.);
#22534=ORIENTED_EDGE('',*,*,#17201,.T.);
#22535=ORIENTED_EDGE('',*,*,#17206,.T.);
#22536=ORIENTED_EDGE('',*,*,#17207,.F.);
#22537=ORIENTED_EDGE('',*,*,#17206,.F.);
#22538=ORIENTED_EDGE('',*,*,#17200,.F.);
#22539=ORIENTED_EDGE('',*,*,#17208,.F.);
#22540=ORIENTED_EDGE('',*,*,#17209,.T.);
#22541=ORIENTED_EDGE('',*,*,#17210,.F.);
#22542=ORIENTED_EDGE('',*,*,#17211,.T.);
#22543=ORIENTED_EDGE('',*,*,#17212,.F.);
#22544=ORIENTED_EDGE('',*,*,#17211,.F.);
#22545=ORIENTED_EDGE('',*,*,#17213,.F.);
#22546=ORIENTED_EDGE('',*,*,#17214,.F.);
#22547=ORIENTED_EDGE('',*,*,#17213,.T.);
#22548=ORIENTED_EDGE('',*,*,#17210,.T.);
#22549=ORIENTED_EDGE('',*,*,#17215,.T.);
#22550=ORIENTED_EDGE('',*,*,#17216,.F.);
#22551=ORIENTED_EDGE('',*,*,#17215,.F.);
#22552=ORIENTED_EDGE('',*,*,#17209,.F.);
#22553=ORIENTED_EDGE('',*,*,#16849,.T.);
#22554=ORIENTED_EDGE('',*,*,#17217,.F.);
#22555=ORIENTED_EDGE('',*,*,#17218,.T.);
#22556=ORIENTED_EDGE('',*,*,#17219,.F.);
#22557=ORIENTED_EDGE('',*,*,#17220,.F.);
#22558=ORIENTED_EDGE('',*,*,#16858,.F.);
#22559=ORIENTED_EDGE('',*,*,#16856,.F.);
#22560=ORIENTED_EDGE('',*,*,#16850,.T.);
#22561=ORIENTED_EDGE('',*,*,#17219,.T.);
#22562=ORIENTED_EDGE('',*,*,#17221,.T.);
#22563=ORIENTED_EDGE('',*,*,#17222,.F.);
#22564=ORIENTED_EDGE('',*,*,#17223,.F.);
#22565=ORIENTED_EDGE('',*,*,#17221,.F.);
#22566=ORIENTED_EDGE('',*,*,#17218,.F.);
#22567=ORIENTED_EDGE('',*,*,#17224,.F.);
#22568=ORIENTED_EDGE('',*,*,#16876,.F.);
#22569=ORIENTED_EDGE('',*,*,#16871,.F.);
#22570=ORIENTED_EDGE('',*,*,#17225,.F.);
#22571=ORIENTED_EDGE('',*,*,#16874,.F.);
#22572=ORIENTED_EDGE('',*,*,#16879,.F.);
#22573=ORIENTED_EDGE('',*,*,#17226,.F.);
#22574=ORIENTED_EDGE('',*,*,#17227,.T.);
#22575=ORIENTED_EDGE('',*,*,#17228,.F.);
#22576=ORIENTED_EDGE('',*,*,#17227,.F.);
#22577=ORIENTED_EDGE('',*,*,#17229,.F.);
#22578=ORIENTED_EDGE('',*,*,#17228,.T.);
#22579=ORIENTED_EDGE('',*,*,#17230,.F.);
#22580=ORIENTED_EDGE('',*,*,#17231,.T.);
#22581=ORIENTED_EDGE('',*,*,#17229,.T.);
#22582=ORIENTED_EDGE('',*,*,#17231,.F.);
#22583=ORIENTED_EDGE('',*,*,#17232,.F.);
#22584=ORIENTED_EDGE('',*,*,#17233,.T.);
#22585=ORIENTED_EDGE('',*,*,#17050,.T.);
#22586=ORIENTED_EDGE('',*,*,#17051,.T.);
#22587=ORIENTED_EDGE('',*,*,#17053,.T.);
#22588=ORIENTED_EDGE('',*,*,#17234,.T.);
#22589=ORIENTED_EDGE('',*,*,#17230,.T.);
#22590=ORIENTED_EDGE('',*,*,#17234,.F.);
#22591=ORIENTED_EDGE('',*,*,#17054,.T.);
#22592=ORIENTED_EDGE('',*,*,#17044,.T.);
#22593=ORIENTED_EDGE('',*,*,#17048,.T.);
#22594=ORIENTED_EDGE('',*,*,#17233,.F.);
#22595=ORIENTED_EDGE('',*,*,#16848,.T.);
#22596=ORIENTED_EDGE('',*,*,#16875,.T.);
#22597=ORIENTED_EDGE('',*,*,#17225,.T.);
#22598=ORIENTED_EDGE('',*,*,#16878,.T.);
#22599=ORIENTED_EDGE('',*,*,#16845,.T.);
#22600=ORIENTED_EDGE('',*,*,#16869,.T.);
#22601=ORIENTED_EDGE('',*,*,#16881,.T.);
#22602=ORIENTED_EDGE('',*,*,#16863,.T.);
#22603=ORIENTED_EDGE('',*,*,#16842,.T.);
#22604=ORIENTED_EDGE('',*,*,#16862,.T.);
#22605=ORIENTED_EDGE('',*,*,#16880,.T.);
#22606=ORIENTED_EDGE('',*,*,#16866,.T.);
#22607=ORIENTED_EDGE('',*,*,#16839,.T.);
#22608=ORIENTED_EDGE('',*,*,#16877,.T.);
#22609=ORIENTED_EDGE('',*,*,#17224,.T.);
#22610=ORIENTED_EDGE('',*,*,#16870,.T.);
#22611=ORIENTED_EDGE('',*,*,#16836,.T.);
#22612=ORIENTED_EDGE('',*,*,#16859,.T.);
#22613=ORIENTED_EDGE('',*,*,#17220,.T.);
#22614=ORIENTED_EDGE('',*,*,#16855,.T.);
#22615=ORIENTED_EDGE('',*,*,#16833,.T.);
#22616=ORIENTED_EDGE('',*,*,#16851,.T.);
#22617=ORIENTED_EDGE('',*,*,#17222,.T.);
#22618=ORIENTED_EDGE('',*,*,#17223,.T.);
#22619=ORIENTED_EDGE('',*,*,#17217,.T.);
#22620=ORIENTED_EDGE('',*,*,#16888,.T.);
#22621=ORIENTED_EDGE('',*,*,#16890,.T.);
#22622=ORIENTED_EDGE('',*,*,#16882,.T.);
#22623=ORIENTED_EDGE('',*,*,#16886,.T.);
#22624=ORIENTED_EDGE('',*,*,#16897,.T.);
#22625=ORIENTED_EDGE('',*,*,#16899,.T.);
#22626=ORIENTED_EDGE('',*,*,#16891,.T.);
#22627=ORIENTED_EDGE('',*,*,#16895,.T.);
#22628=ORIENTED_EDGE('',*,*,#16906,.T.);
#22629=ORIENTED_EDGE('',*,*,#16908,.T.);
#22630=ORIENTED_EDGE('',*,*,#16900,.T.);
#22631=ORIENTED_EDGE('',*,*,#16904,.T.);
#22632=ORIENTED_EDGE('',*,*,#16915,.T.);
#22633=ORIENTED_EDGE('',*,*,#16917,.T.);
#22634=ORIENTED_EDGE('',*,*,#16909,.T.);
#22635=ORIENTED_EDGE('',*,*,#16913,.T.);
#22636=ORIENTED_EDGE('',*,*,#16924,.T.);
#22637=ORIENTED_EDGE('',*,*,#16926,.T.);
#22638=ORIENTED_EDGE('',*,*,#16918,.T.);
#22639=ORIENTED_EDGE('',*,*,#16922,.T.);
#22640=ORIENTED_EDGE('',*,*,#16933,.T.);
#22641=ORIENTED_EDGE('',*,*,#16935,.T.);
#22642=ORIENTED_EDGE('',*,*,#16927,.T.);
#22643=ORIENTED_EDGE('',*,*,#16931,.T.);
#22644=ORIENTED_EDGE('',*,*,#16942,.T.);
#22645=ORIENTED_EDGE('',*,*,#16944,.T.);
#22646=ORIENTED_EDGE('',*,*,#16936,.T.);
#22647=ORIENTED_EDGE('',*,*,#16940,.T.);
#22648=ORIENTED_EDGE('',*,*,#16951,.T.);
#22649=ORIENTED_EDGE('',*,*,#16953,.T.);
#22650=ORIENTED_EDGE('',*,*,#16945,.T.);
#22651=ORIENTED_EDGE('',*,*,#16949,.T.);
#22652=ORIENTED_EDGE('',*,*,#16960,.T.);
#22653=ORIENTED_EDGE('',*,*,#16962,.T.);
#22654=ORIENTED_EDGE('',*,*,#16954,.T.);
#22655=ORIENTED_EDGE('',*,*,#16958,.T.);
#22656=ORIENTED_EDGE('',*,*,#16969,.T.);
#22657=ORIENTED_EDGE('',*,*,#16971,.T.);
#22658=ORIENTED_EDGE('',*,*,#16963,.T.);
#22659=ORIENTED_EDGE('',*,*,#16967,.T.);
#22660=ORIENTED_EDGE('',*,*,#16978,.T.);
#22661=ORIENTED_EDGE('',*,*,#16980,.T.);
#22662=ORIENTED_EDGE('',*,*,#16972,.T.);
#22663=ORIENTED_EDGE('',*,*,#16976,.T.);
#22664=ORIENTED_EDGE('',*,*,#16987,.T.);
#22665=ORIENTED_EDGE('',*,*,#16989,.T.);
#22666=ORIENTED_EDGE('',*,*,#16981,.T.);
#22667=ORIENTED_EDGE('',*,*,#16985,.T.);
#22668=ORIENTED_EDGE('',*,*,#16996,.T.);
#22669=ORIENTED_EDGE('',*,*,#16998,.T.);
#22670=ORIENTED_EDGE('',*,*,#16990,.T.);
#22671=ORIENTED_EDGE('',*,*,#16994,.T.);
#22672=ORIENTED_EDGE('',*,*,#17005,.T.);
#22673=ORIENTED_EDGE('',*,*,#17007,.T.);
#22674=ORIENTED_EDGE('',*,*,#16999,.T.);
#22675=ORIENTED_EDGE('',*,*,#17003,.T.);
#22676=ORIENTED_EDGE('',*,*,#17014,.T.);
#22677=ORIENTED_EDGE('',*,*,#17016,.T.);
#22678=ORIENTED_EDGE('',*,*,#17008,.T.);
#22679=ORIENTED_EDGE('',*,*,#17012,.T.);
#22680=ORIENTED_EDGE('',*,*,#17023,.T.);
#22681=ORIENTED_EDGE('',*,*,#17025,.T.);
#22682=ORIENTED_EDGE('',*,*,#17017,.T.);
#22683=ORIENTED_EDGE('',*,*,#17021,.T.);
#22684=ORIENTED_EDGE('',*,*,#17032,.T.);
#22685=ORIENTED_EDGE('',*,*,#17034,.T.);
#22686=ORIENTED_EDGE('',*,*,#17026,.T.);
#22687=ORIENTED_EDGE('',*,*,#17030,.T.);
#22688=ORIENTED_EDGE('',*,*,#17041,.T.);
#22689=ORIENTED_EDGE('',*,*,#17043,.T.);
#22690=ORIENTED_EDGE('',*,*,#17035,.T.);
#22691=ORIENTED_EDGE('',*,*,#17039,.T.);
#22692=ORIENTED_EDGE('',*,*,#17061,.T.);
#22693=ORIENTED_EDGE('',*,*,#17063,.T.);
#22694=ORIENTED_EDGE('',*,*,#17055,.T.);
#22695=ORIENTED_EDGE('',*,*,#17059,.T.);
#22696=ORIENTED_EDGE('',*,*,#17070,.T.);
#22697=ORIENTED_EDGE('',*,*,#17072,.T.);
#22698=ORIENTED_EDGE('',*,*,#17064,.T.);
#22699=ORIENTED_EDGE('',*,*,#17068,.T.);
#22700=ORIENTED_EDGE('',*,*,#17079,.T.);
#22701=ORIENTED_EDGE('',*,*,#17081,.T.);
#22702=ORIENTED_EDGE('',*,*,#17073,.T.);
#22703=ORIENTED_EDGE('',*,*,#17077,.T.);
#22704=ORIENTED_EDGE('',*,*,#17088,.T.);
#22705=ORIENTED_EDGE('',*,*,#17090,.T.);
#22706=ORIENTED_EDGE('',*,*,#17082,.T.);
#22707=ORIENTED_EDGE('',*,*,#17086,.T.);
#22708=ORIENTED_EDGE('',*,*,#17097,.T.);
#22709=ORIENTED_EDGE('',*,*,#17099,.T.);
#22710=ORIENTED_EDGE('',*,*,#17091,.T.);
#22711=ORIENTED_EDGE('',*,*,#17095,.T.);
#22712=ORIENTED_EDGE('',*,*,#17106,.T.);
#22713=ORIENTED_EDGE('',*,*,#17108,.T.);
#22714=ORIENTED_EDGE('',*,*,#17100,.T.);
#22715=ORIENTED_EDGE('',*,*,#17104,.T.);
#22716=ORIENTED_EDGE('',*,*,#17115,.T.);
#22717=ORIENTED_EDGE('',*,*,#17117,.T.);
#22718=ORIENTED_EDGE('',*,*,#17109,.T.);
#22719=ORIENTED_EDGE('',*,*,#17113,.T.);
#22720=ORIENTED_EDGE('',*,*,#17124,.T.);
#22721=ORIENTED_EDGE('',*,*,#17126,.T.);
#22722=ORIENTED_EDGE('',*,*,#17118,.T.);
#22723=ORIENTED_EDGE('',*,*,#17122,.T.);
#22724=ORIENTED_EDGE('',*,*,#17133,.T.);
#22725=ORIENTED_EDGE('',*,*,#17135,.T.);
#22726=ORIENTED_EDGE('',*,*,#17127,.T.);
#22727=ORIENTED_EDGE('',*,*,#17131,.T.);
#22728=ORIENTED_EDGE('',*,*,#17142,.T.);
#22729=ORIENTED_EDGE('',*,*,#17144,.T.);
#22730=ORIENTED_EDGE('',*,*,#17136,.T.);
#22731=ORIENTED_EDGE('',*,*,#17140,.T.);
#22732=ORIENTED_EDGE('',*,*,#17151,.T.);
#22733=ORIENTED_EDGE('',*,*,#17153,.T.);
#22734=ORIENTED_EDGE('',*,*,#17145,.T.);
#22735=ORIENTED_EDGE('',*,*,#17149,.T.);
#22736=ORIENTED_EDGE('',*,*,#17160,.T.);
#22737=ORIENTED_EDGE('',*,*,#17162,.T.);
#22738=ORIENTED_EDGE('',*,*,#17154,.T.);
#22739=ORIENTED_EDGE('',*,*,#17158,.T.);
#22740=ORIENTED_EDGE('',*,*,#17169,.T.);
#22741=ORIENTED_EDGE('',*,*,#17171,.T.);
#22742=ORIENTED_EDGE('',*,*,#17163,.T.);
#22743=ORIENTED_EDGE('',*,*,#17167,.T.);
#22744=ORIENTED_EDGE('',*,*,#17178,.T.);
#22745=ORIENTED_EDGE('',*,*,#17180,.T.);
#22746=ORIENTED_EDGE('',*,*,#17172,.T.);
#22747=ORIENTED_EDGE('',*,*,#17176,.T.);
#22748=ORIENTED_EDGE('',*,*,#17187,.T.);
#22749=ORIENTED_EDGE('',*,*,#17189,.T.);
#22750=ORIENTED_EDGE('',*,*,#17181,.T.);
#22751=ORIENTED_EDGE('',*,*,#17185,.T.);
#22752=ORIENTED_EDGE('',*,*,#17196,.T.);
#22753=ORIENTED_EDGE('',*,*,#17198,.T.);
#22754=ORIENTED_EDGE('',*,*,#17190,.T.);
#22755=ORIENTED_EDGE('',*,*,#17194,.T.);
#22756=ORIENTED_EDGE('',*,*,#17205,.T.);
#22757=ORIENTED_EDGE('',*,*,#17207,.T.);
#22758=ORIENTED_EDGE('',*,*,#17199,.T.);
#22759=ORIENTED_EDGE('',*,*,#17203,.T.);
#22760=ORIENTED_EDGE('',*,*,#17214,.T.);
#22761=ORIENTED_EDGE('',*,*,#17216,.T.);
#22762=ORIENTED_EDGE('',*,*,#17208,.T.);
#22763=ORIENTED_EDGE('',*,*,#17212,.T.);
#22764=ORIENTED_EDGE('',*,*,#17232,.T.);
#22765=ORIENTED_EDGE('',*,*,#17235,.T.);
#22766=ORIENTED_EDGE('',*,*,#17236,.F.);
#22767=ORIENTED_EDGE('',*,*,#17235,.F.);
#22768=ORIENTED_EDGE('',*,*,#17236,.T.);
#22769=ORIENTED_EDGE('',*,*,#17237,.F.);
#22770=ORIENTED_EDGE('',*,*,#17238,.F.);
#22771=ORIENTED_EDGE('',*,*,#17239,.T.);
#22772=ORIENTED_EDGE('',*,*,#17237,.T.);
#22773=ORIENTED_EDGE('',*,*,#17239,.F.);
#22774=ORIENTED_EDGE('',*,*,#17238,.T.);
#22775=ORIENTED_EDGE('',*,*,#17240,.F.);
#22776=ORIENTED_EDGE('',*,*,#17226,.T.);
#22777=ORIENTED_EDGE('',*,*,#17241,.T.);
#22778=ORIENTED_EDGE('',*,*,#17240,.T.);
#22779=ORIENTED_EDGE('',*,*,#17241,.F.);
#22780=ORIENTED_EDGE('',*,*,#16853,.T.);
#22781=ORIENTED_EDGE('',*,*,#16854,.T.);
#30289=CONICAL_SURFACE('',#32739,3.905,1.43962768039283);
#30290=CONICAL_SURFACE('',#32744,7.2,0.785398163397444);
#30291=CONICAL_SURFACE('',#32748,7.3,0.785398163397437);
#30507=ADVANCED_FACE('',(#3532),#1836,.F.);
#30508=ADVANCED_FACE('',(#3533),#2281,.F.);
#30509=ADVANCED_FACE('',(#3534),#2282,.F.);
#30510=ADVANCED_FACE('',(#3535),#2283,.F.);
#30511=ADVANCED_FACE('',(#3536),#2284,.F.);
#30512=ADVANCED_FACE('',(#3537),#2285,.F.);
#30513=ADVANCED_FACE('',(#3538),#2286,.F.);
#30514=ADVANCED_FACE('',(#3539),#2287,.F.);
#30515=ADVANCED_FACE('',(#3540),#2288,.F.);
#30516=ADVANCED_FACE('',(#3541),#2289,.F.);
#30517=ADVANCED_FACE('',(#3542),#2290,.F.);
#30518=ADVANCED_FACE('',(#3543),#2291,.T.);
#30519=ADVANCED_FACE('',(#3544),#2292,.F.);
#30520=ADVANCED_FACE('',(#3545),#2293,.F.);
#30521=ADVANCED_FACE('',(#3546),#2294,.T.);
#30522=ADVANCED_FACE('',(#3547),#2295,.F.);
#30523=ADVANCED_FACE('',(#3548),#2296,.F.);
#30524=ADVANCED_FACE('',(#3549),#2297,.F.);
#30525=ADVANCED_FACE('',(#3550),#2298,.T.);
#30526=ADVANCED_FACE('',(#3551),#2299,.F.);
#30527=ADVANCED_FACE('',(#3552),#2300,.F.);
#30528=ADVANCED_FACE('',(#3553),#2301,.F.);
#30529=ADVANCED_FACE('',(#3554),#2302,.T.);
#30530=ADVANCED_FACE('',(#3555),#2303,.F.);
#30531=ADVANCED_FACE('',(#3556),#2304,.F.);
#30532=ADVANCED_FACE('',(#3557),#2305,.F.);
#30533=ADVANCED_FACE('',(#3558),#2306,.T.);
#30534=ADVANCED_FACE('',(#3559),#2307,.F.);
#30535=ADVANCED_FACE('',(#3560),#2308,.F.);
#30536=ADVANCED_FACE('',(#3561),#2309,.F.);
#30537=ADVANCED_FACE('',(#3562),#2310,.T.);
#30538=ADVANCED_FACE('',(#3563),#2311,.F.);
#30539=ADVANCED_FACE('',(#3564),#2312,.F.);
#30540=ADVANCED_FACE('',(#3565),#2313,.F.);
#30541=ADVANCED_FACE('',(#3566),#2314,.T.);
#30542=ADVANCED_FACE('',(#3567),#2315,.F.);
#30543=ADVANCED_FACE('',(#3568),#2316,.F.);
#30544=ADVANCED_FACE('',(#3569),#2317,.F.);
#30545=ADVANCED_FACE('',(#3570),#2318,.T.);
#30546=ADVANCED_FACE('',(#3571),#2319,.F.);
#30547=ADVANCED_FACE('',(#3572),#2320,.F.);
#30548=ADVANCED_FACE('',(#3573),#2321,.F.);
#30549=ADVANCED_FACE('',(#3574),#2322,.T.);
#30550=ADVANCED_FACE('',(#3575),#2323,.F.);
#30551=ADVANCED_FACE('',(#3576),#2324,.F.);
#30552=ADVANCED_FACE('',(#3577),#2325,.F.);
#30553=ADVANCED_FACE('',(#3578),#2326,.T.);
#30554=ADVANCED_FACE('',(#3579),#2327,.F.);
#30555=ADVANCED_FACE('',(#3580),#2328,.F.);
#30556=ADVANCED_FACE('',(#3581),#2329,.F.);
#30557=ADVANCED_FACE('',(#3582),#2330,.T.);
#30558=ADVANCED_FACE('',(#3583),#2331,.F.);
#30559=ADVANCED_FACE('',(#3584),#2332,.F.);
#30560=ADVANCED_FACE('',(#3585),#2333,.F.);
#30561=ADVANCED_FACE('',(#3586),#2334,.T.);
#30562=ADVANCED_FACE('',(#3587),#2335,.F.);
#30563=ADVANCED_FACE('',(#3588),#2336,.F.);
#30564=ADVANCED_FACE('',(#3589),#2337,.F.);
#30565=ADVANCED_FACE('',(#3590),#2338,.T.);
#30566=ADVANCED_FACE('',(#3591),#2339,.F.);
#30567=ADVANCED_FACE('',(#3592),#2340,.F.);
#30568=ADVANCED_FACE('',(#3593),#2341,.F.);
#30569=ADVANCED_FACE('',(#3594),#2342,.T.);
#30570=ADVANCED_FACE('',(#3595),#2343,.F.);
#30571=ADVANCED_FACE('',(#3596),#2344,.F.);
#30572=ADVANCED_FACE('',(#3597),#2345,.F.);
#30573=ADVANCED_FACE('',(#3598),#2346,.T.);
#30574=ADVANCED_FACE('',(#3599),#2347,.F.);
#30575=ADVANCED_FACE('',(#3600),#2348,.F.);
#30576=ADVANCED_FACE('',(#3601),#2349,.F.);
#30577=ADVANCED_FACE('',(#3602),#2350,.T.);
#30578=ADVANCED_FACE('',(#3603),#2351,.F.);
#30579=ADVANCED_FACE('',(#3604),#2352,.F.);
#30580=ADVANCED_FACE('',(#3605),#2353,.F.);
#30581=ADVANCED_FACE('',(#3606),#2354,.T.);
#30582=ADVANCED_FACE('',(#3607),#2355,.F.);
#30583=ADVANCED_FACE('',(#3608),#2356,.F.);
#30584=ADVANCED_FACE('',(#3609),#2357,.F.);
#30585=ADVANCED_FACE('',(#3610),#2358,.T.);
#30586=ADVANCED_FACE('',(#3611),#2359,.F.);
#30587=ADVANCED_FACE('',(#3612),#2360,.F.);
#30588=ADVANCED_FACE('',(#3613),#2361,.F.);
#30589=ADVANCED_FACE('',(#3614),#2362,.T.);
#30590=ADVANCED_FACE('',(#3615),#2363,.F.);
#30591=ADVANCED_FACE('',(#3616),#2364,.F.);
#30592=ADVANCED_FACE('',(#3617),#2365,.F.);
#30593=ADVANCED_FACE('',(#3618),#2366,.T.);
#30594=ADVANCED_FACE('',(#3619),#2367,.F.);
#30595=ADVANCED_FACE('',(#3620),#2368,.F.);
#30596=ADVANCED_FACE('',(#3621),#2369,.F.);
#30597=ADVANCED_FACE('',(#3622),#2370,.T.);
#30598=ADVANCED_FACE('',(#3623),#2371,.F.);
#30599=ADVANCED_FACE('',(#3624),#2372,.F.);
#30600=ADVANCED_FACE('',(#3625),#2373,.F.);
#30601=ADVANCED_FACE('',(#3626),#2374,.T.);
#30602=ADVANCED_FACE('',(#3627),#2375,.F.);
#30603=ADVANCED_FACE('',(#3628),#2376,.F.);
#30604=ADVANCED_FACE('',(#3629),#2377,.F.);
#30605=ADVANCED_FACE('',(#3630),#2378,.T.);
#30606=ADVANCED_FACE('',(#3631),#2379,.F.);
#30607=ADVANCED_FACE('',(#3632),#2380,.F.);
#30608=ADVANCED_FACE('',(#3633),#2381,.F.);
#30609=ADVANCED_FACE('',(#3634),#2382,.T.);
#30610=ADVANCED_FACE('',(#3635),#2383,.F.);
#30611=ADVANCED_FACE('',(#3636),#2384,.F.);
#30612=ADVANCED_FACE('',(#3637),#2385,.F.);
#30613=ADVANCED_FACE('',(#3638),#2386,.T.);
#30614=ADVANCED_FACE('',(#3639),#2387,.F.);
#30615=ADVANCED_FACE('',(#3640),#2388,.F.);
#30616=ADVANCED_FACE('',(#3641),#2389,.F.);
#30617=ADVANCED_FACE('',(#3642),#2390,.T.);
#30618=ADVANCED_FACE('',(#3643),#2391,.F.);
#30619=ADVANCED_FACE('',(#3644),#2392,.F.);
#30620=ADVANCED_FACE('',(#3645),#2393,.F.);
#30621=ADVANCED_FACE('',(#3646),#2394,.T.);
#30622=ADVANCED_FACE('',(#3647),#2395,.F.);
#30623=ADVANCED_FACE('',(#3648),#2396,.F.);
#30624=ADVANCED_FACE('',(#3649),#2397,.F.);
#30625=ADVANCED_FACE('',(#3650),#2398,.T.);
#30626=ADVANCED_FACE('',(#3651),#2399,.F.);
#30627=ADVANCED_FACE('',(#3652),#2400,.F.);
#30628=ADVANCED_FACE('',(#3653),#2401,.F.);
#30629=ADVANCED_FACE('',(#3654),#2402,.T.);
#30630=ADVANCED_FACE('',(#3655),#2403,.F.);
#30631=ADVANCED_FACE('',(#3656),#2404,.F.);
#30632=ADVANCED_FACE('',(#3657),#2405,.F.);
#30633=ADVANCED_FACE('',(#3658),#2406,.T.);
#30634=ADVANCED_FACE('',(#3659),#2407,.F.);
#30635=ADVANCED_FACE('',(#3660),#2408,.F.);
#30636=ADVANCED_FACE('',(#3661),#2409,.F.);
#30637=ADVANCED_FACE('',(#3662),#2410,.T.);
#30638=ADVANCED_FACE('',(#3663),#2411,.F.);
#30639=ADVANCED_FACE('',(#3664),#2412,.F.);
#30640=ADVANCED_FACE('',(#3665),#2413,.F.);
#30641=ADVANCED_FACE('',(#3666),#2414,.T.);
#30642=ADVANCED_FACE('',(#3667),#2415,.F.);
#30643=ADVANCED_FACE('',(#3668),#2416,.F.);
#30644=ADVANCED_FACE('',(#3669),#2417,.F.);
#30645=ADVANCED_FACE('',(#3670),#2418,.T.);
#30646=ADVANCED_FACE('',(#3671),#2419,.F.);
#30647=ADVANCED_FACE('',(#3672),#2420,.F.);
#30648=ADVANCED_FACE('',(#3673),#2421,.F.);
#30649=ADVANCED_FACE('',(#3674),#2422,.T.);
#30650=ADVANCED_FACE('',(#3675),#2423,.F.);
#30651=ADVANCED_FACE('',(#3676),#2424,.F.);
#30652=ADVANCED_FACE('',(#3677),#2425,.F.);
#30653=ADVANCED_FACE('',(#3678),#2426,.T.);
#30654=ADVANCED_FACE('',(#3679),#2427,.F.);
#30655=ADVANCED_FACE('',(#3680),#2428,.F.);
#30656=ADVANCED_FACE('',(#3681),#2429,.F.);
#30657=ADVANCED_FACE('',(#3682),#2430,.T.);
#30658=ADVANCED_FACE('',(#3683),#2431,.F.);
#30659=ADVANCED_FACE('',(#3684),#2432,.F.);
#30660=ADVANCED_FACE('',(#3685),#2433,.F.);
#30661=ADVANCED_FACE('',(#3686),#2434,.T.);
#30662=ADVANCED_FACE('',(#3687),#2435,.F.);
#30663=ADVANCED_FACE('',(#3688),#2436,.F.);
#30664=ADVANCED_FACE('',(#3689),#2437,.F.);
#30665=ADVANCED_FACE('',(#3690),#2438,.T.);
#30666=ADVANCED_FACE('',(#3691),#2439,.F.);
#30667=ADVANCED_FACE('',(#3692),#2440,.F.);
#30668=ADVANCED_FACE('',(#3693),#2441,.F.);
#30669=ADVANCED_FACE('',(#3694),#2442,.T.);
#30670=ADVANCED_FACE('',(#3695),#2443,.F.);
#30671=ADVANCED_FACE('',(#3696),#2444,.F.);
#30672=ADVANCED_FACE('',(#3697),#2445,.T.);
#30673=ADVANCED_FACE('',(#3698),#2446,.F.);
#30674=ADVANCED_FACE('',(#3699),#30289,.F.);
#30675=ADVANCED_FACE('',(#3700,#2037),#2447,.T.);
#30676=ADVANCED_FACE('',(#3701),#30290,.T.);
#30677=ADVANCED_FACE('',(#3702,#2038,#2039,#2040,#2041,#2042,#2043,#2044,
#2045,#2046,#2047,#2048,#2049,#2050,#2051,#2052,#2053,#2054,#2055,#2056,
#2057,#2058,#2059,#2060,#2061,#2062,#2063,#2064,#2065,#2066,#2067,#2068,
#2069,#2070,#2071,#2072,#2073,#2074),#1837,.T.);
#30678=ADVANCED_FACE('',(#3703),#30291,.T.);
#30679=ADVANCED_FACE('',(#3704,#2075),#2448,.T.);
#30680=ADVANCED_FACE('',(#3705),#1838,.T.);
#30681=ADVANCED_FACE('',(#3706,#2076),#2449,.T.);
#30682=ADVANCED_FACE('',(#3707,#2077),#1839,.F.);
#32079=CLOSED_SHELL('',(#30507,#30508,#30509,#30510,#30511,#30512,#30513,
#30514,#30515,#30516,#30517,#30518,#30519,#30520,#30521,#30522,#30523,#30524,
#30525,#30526,#30527,#30528,#30529,#30530,#30531,#30532,#30533,#30534,#30535,
#30536,#30537,#30538,#30539,#30540,#30541,#30542,#30543,#30544,#30545,#30546,
#30547,#30548,#30549,#30550,#30551,#30552,#30553,#30554,#30555,#30556,#30557,
#30558,#30559,#30560,#30561,#30562,#30563,#30564,#30565,#30566,#30567,#30568,
#30569,#30570,#30571,#30572,#30573,#30574,#30575,#30576,#30577,#30578,#30579,
#30580,#30581,#30582,#30583,#30584,#30585,#30586,#30587,#30588,#30589,#30590,
#30591,#30592,#30593,#30594,#30595,#30596,#30597,#30598,#30599,#30600,#30601,
#30602,#30603,#30604,#30605,#30606,#30607,#30608,#30609,#30610,#30611,#30612,
#30613,#30614,#30615,#30616,#30617,#30618,#30619,#30620,#30621,#30622,#30623,
#30624,#30625,#30626,#30627,#30628,#30629,#30630,#30631,#30632,#30633,#30634,
#30635,#30636,#30637,#30638,#30639,#30640,#30641,#30642,#30643,#30644,#30645,
#30646,#30647,#30648,#30649,#30650,#30651,#30652,#30653,#30654,#30655,#30656,
#30657,#30658,#30659,#30660,#30661,#30662,#30663,#30664,#30665,#30666,#30667,
#30668,#30669,#30670,#30671,#30672,#30673,#30674,#30675,#30676,#30677,#30678,
#30679,#30680,#30681,#30682));
#32477=AXIS2_PLACEMENT_3D('',#69010,#34933,#34934);
#32478=AXIS2_PLACEMENT_3D('',#69011,#34935,#34936);
#32479=AXIS2_PLACEMENT_3D('',#69021,#34937,#34938);
#32480=AXIS2_PLACEMENT_3D('',#69023,#34939,#34940);
#32481=AXIS2_PLACEMENT_3D('',#69032,#34941,#34942);
#32482=AXIS2_PLACEMENT_3D('',#69034,#34943,#34944);
#32483=AXIS2_PLACEMENT_3D('',#69043,#34945,#34946);
#32484=AXIS2_PLACEMENT_3D('',#69045,#34947,#34948);
#32485=AXIS2_PLACEMENT_3D('',#69059,#34949,#34950);
#32486=AXIS2_PLACEMENT_3D('',#69061,#34951,#34952);
#32487=AXIS2_PLACEMENT_3D('',#69070,#34953,#34954);
#32488=AXIS2_PLACEMENT_3D('',#69072,#34955,#34956);
#32489=AXIS2_PLACEMENT_3D('',#69081,#34957,#34958);
#32490=AXIS2_PLACEMENT_3D('',#69083,#34959,#34960);
#32491=AXIS2_PLACEMENT_3D('',#69137,#34962,#34963);
#32492=AXIS2_PLACEMENT_3D('',#69143,#34967,#34968);
#32493=AXIS2_PLACEMENT_3D('',#69147,#34971,#34972);
#32494=AXIS2_PLACEMENT_3D('',#69153,#34976,#34977);
#32495=AXIS2_PLACEMENT_3D('',#69159,#34981,#34982);
#32496=AXIS2_PLACEMENT_3D('',#69163,#34985,#34986);
#32497=AXIS2_PLACEMENT_3D('',#69167,#34989,#34990);
#32498=AXIS2_PLACEMENT_3D('',#69173,#34994,#34995);
#32499=AXIS2_PLACEMENT_3D('',#69179,#34999,#35000);
#32500=AXIS2_PLACEMENT_3D('',#69183,#35003,#35004);
#32501=AXIS2_PLACEMENT_3D('',#69187,#35007,#35008);
#32502=AXIS2_PLACEMENT_3D('',#69188,#35009,#35010);
#32503=AXIS2_PLACEMENT_3D('',#69189,#35011,#35012);
#32504=AXIS2_PLACEMENT_3D('',#69190,#35013,#35014);
#32505=AXIS2_PLACEMENT_3D('',#69191,#35015,#35016);
#32506=AXIS2_PLACEMENT_3D('',#69200,#35021,#35022);
#32507=AXIS2_PLACEMENT_3D('',#69202,#35023,#35024);
#32508=AXIS2_PLACEMENT_3D('',#69204,#35026,#35027);
#32509=AXIS2_PLACEMENT_3D('',#69208,#35030,#35031);
#32510=AXIS2_PLACEMENT_3D('',#69209,#35032,#35033);
#32511=AXIS2_PLACEMENT_3D('',#69210,#35034,#35035);
#32512=AXIS2_PLACEMENT_3D('',#69219,#35040,#35041);
#32513=AXIS2_PLACEMENT_3D('',#69221,#35042,#35043);
#32514=AXIS2_PLACEMENT_3D('',#69223,#35045,#35046);
#32515=AXIS2_PLACEMENT_3D('',#69227,#35049,#35050);
#32516=AXIS2_PLACEMENT_3D('',#69228,#35051,#35052);
#32517=AXIS2_PLACEMENT_3D('',#69229,#35053,#35054);
#32518=AXIS2_PLACEMENT_3D('',#69238,#35059,#35060);
#32519=AXIS2_PLACEMENT_3D('',#69240,#35061,#35062);
#32520=AXIS2_PLACEMENT_3D('',#69242,#35064,#35065);
#32521=AXIS2_PLACEMENT_3D('',#69246,#35068,#35069);
#32522=AXIS2_PLACEMENT_3D('',#69247,#35070,#35071);
#32523=AXIS2_PLACEMENT_3D('',#69248,#35072,#35073);
#32524=AXIS2_PLACEMENT_3D('',#69257,#35078,#35079);
#32525=AXIS2_PLACEMENT_3D('',#69259,#35080,#35081);
#32526=AXIS2_PLACEMENT_3D('',#69261,#35083,#35084);
#32527=AXIS2_PLACEMENT_3D('',#69265,#35087,#35088);
#32528=AXIS2_PLACEMENT_3D('',#69266,#35089,#35090);
#32529=AXIS2_PLACEMENT_3D('',#69267,#35091,#35092);
#32530=AXIS2_PLACEMENT_3D('',#69276,#35097,#35098);
#32531=AXIS2_PLACEMENT_3D('',#69278,#35099,#35100);
#32532=AXIS2_PLACEMENT_3D('',#69280,#35102,#35103);
#32533=AXIS2_PLACEMENT_3D('',#69284,#35106,#35107);
#32534=AXIS2_PLACEMENT_3D('',#69285,#35108,#35109);
#32535=AXIS2_PLACEMENT_3D('',#69286,#35110,#35111);
#32536=AXIS2_PLACEMENT_3D('',#69295,#35116,#35117);
#32537=AXIS2_PLACEMENT_3D('',#69297,#35118,#35119);
#32538=AXIS2_PLACEMENT_3D('',#69299,#35121,#35122);
#32539=AXIS2_PLACEMENT_3D('',#69303,#35125,#35126);
#32540=AXIS2_PLACEMENT_3D('',#69304,#35127,#35128);
#32541=AXIS2_PLACEMENT_3D('',#69305,#35129,#35130);
#32542=AXIS2_PLACEMENT_3D('',#69314,#35135,#35136);
#32543=AXIS2_PLACEMENT_3D('',#69316,#35137,#35138);
#32544=AXIS2_PLACEMENT_3D('',#69318,#35140,#35141);
#32545=AXIS2_PLACEMENT_3D('',#69322,#35144,#35145);
#32546=AXIS2_PLACEMENT_3D('',#69323,#35146,#35147);
#32547=AXIS2_PLACEMENT_3D('',#69324,#35148,#35149);
#32548=AXIS2_PLACEMENT_3D('',#69333,#35154,#35155);
#32549=AXIS2_PLACEMENT_3D('',#69335,#35156,#35157);
#32550=AXIS2_PLACEMENT_3D('',#69337,#35159,#35160);
#32551=AXIS2_PLACEMENT_3D('',#69341,#35163,#35164);
#32552=AXIS2_PLACEMENT_3D('',#69342,#35165,#35166);
#32553=AXIS2_PLACEMENT_3D('',#69343,#35167,#35168);
#32554=AXIS2_PLACEMENT_3D('',#69352,#35173,#35174);
#32555=AXIS2_PLACEMENT_3D('',#69354,#35175,#35176);
#32556=AXIS2_PLACEMENT_3D('',#69356,#35178,#35179);
#32557=AXIS2_PLACEMENT_3D('',#69360,#35182,#35183);
#32558=AXIS2_PLACEMENT_3D('',#69361,#35184,#35185);
#32559=AXIS2_PLACEMENT_3D('',#69362,#35186,#35187);
#32560=AXIS2_PLACEMENT_3D('',#69371,#35192,#35193);
#32561=AXIS2_PLACEMENT_3D('',#69373,#35194,#35195);
#32562=AXIS2_PLACEMENT_3D('',#69375,#35197,#35198);
#32563=AXIS2_PLACEMENT_3D('',#69379,#35201,#35202);
#32564=AXIS2_PLACEMENT_3D('',#69380,#35203,#35204);
#32565=AXIS2_PLACEMENT_3D('',#69381,#35205,#35206);
#32566=AXIS2_PLACEMENT_3D('',#69390,#35211,#35212);
#32567=AXIS2_PLACEMENT_3D('',#69392,#35213,#35214);
#32568=AXIS2_PLACEMENT_3D('',#69394,#35216,#35217);
#32569=AXIS2_PLACEMENT_3D('',#69398,#35220,#35221);
#32570=AXIS2_PLACEMENT_3D('',#69399,#35222,#35223);
#32571=AXIS2_PLACEMENT_3D('',#69400,#35224,#35225);
#32572=AXIS2_PLACEMENT_3D('',#69409,#35230,#35231);
#32573=AXIS2_PLACEMENT_3D('',#69411,#35232,#35233);
#32574=AXIS2_PLACEMENT_3D('',#69413,#35235,#35236);
#32575=AXIS2_PLACEMENT_3D('',#69417,#35239,#35240);
#32576=AXIS2_PLACEMENT_3D('',#69418,#35241,#35242);
#32577=AXIS2_PLACEMENT_3D('',#69419,#35243,#35244);
#32578=AXIS2_PLACEMENT_3D('',#69428,#35249,#35250);
#32579=AXIS2_PLACEMENT_3D('',#69430,#35251,#35252);
#32580=AXIS2_PLACEMENT_3D('',#69432,#35254,#35255);
#32581=AXIS2_PLACEMENT_3D('',#69436,#35258,#35259);
#32582=AXIS2_PLACEMENT_3D('',#69437,#35260,#35261);
#32583=AXIS2_PLACEMENT_3D('',#69438,#35262,#35263);
#32584=AXIS2_PLACEMENT_3D('',#69447,#35268,#35269);
#32585=AXIS2_PLACEMENT_3D('',#69449,#35270,#35271);
#32586=AXIS2_PLACEMENT_3D('',#69451,#35273,#35274);
#32587=AXIS2_PLACEMENT_3D('',#69455,#35277,#35278);
#32588=AXIS2_PLACEMENT_3D('',#69456,#35279,#35280);
#32589=AXIS2_PLACEMENT_3D('',#69457,#35281,#35282);
#32590=AXIS2_PLACEMENT_3D('',#69466,#35287,#35288);
#32591=AXIS2_PLACEMENT_3D('',#69468,#35289,#35290);
#32592=AXIS2_PLACEMENT_3D('',#69470,#35292,#35293);
#32593=AXIS2_PLACEMENT_3D('',#69474,#35296,#35297);
#32594=AXIS2_PLACEMENT_3D('',#69475,#35298,#35299);
#32595=AXIS2_PLACEMENT_3D('',#69476,#35300,#35301);
#32596=AXIS2_PLACEMENT_3D('',#69485,#35306,#35307);
#32597=AXIS2_PLACEMENT_3D('',#69487,#35308,#35309);
#32598=AXIS2_PLACEMENT_3D('',#69489,#35311,#35312);
#32599=AXIS2_PLACEMENT_3D('',#69493,#35315,#35316);
#32600=AXIS2_PLACEMENT_3D('',#69494,#35317,#35318);
#32601=AXIS2_PLACEMENT_3D('',#69495,#35319,#35320);
#32602=AXIS2_PLACEMENT_3D('',#69504,#35325,#35326);
#32603=AXIS2_PLACEMENT_3D('',#69506,#35327,#35328);
#32604=AXIS2_PLACEMENT_3D('',#69508,#35330,#35331);
#32605=AXIS2_PLACEMENT_3D('',#69512,#35334,#35335);
#32606=AXIS2_PLACEMENT_3D('',#69513,#35336,#35337);
#32607=AXIS2_PLACEMENT_3D('',#69514,#35338,#35339);
#32608=AXIS2_PLACEMENT_3D('',#69523,#35344,#35345);
#32609=AXIS2_PLACEMENT_3D('',#69525,#35346,#35347);
#32610=AXIS2_PLACEMENT_3D('',#69527,#35349,#35350);
#32611=AXIS2_PLACEMENT_3D('',#69531,#35353,#35354);
#32612=AXIS2_PLACEMENT_3D('',#69532,#35355,#35356);
#32613=AXIS2_PLACEMENT_3D('',#69533,#35357,#35358);
#32614=AXIS2_PLACEMENT_3D('',#69542,#35363,#35364);
#32615=AXIS2_PLACEMENT_3D('',#69544,#35365,#35366);
#32616=AXIS2_PLACEMENT_3D('',#69547,#35368,#35369);
#32617=AXIS2_PLACEMENT_3D('',#69548,#35370,#35371);
#32618=AXIS2_PLACEMENT_3D('',#69552,#35374,#35375);
#32619=AXIS2_PLACEMENT_3D('',#69554,#35376,#35377);
#32620=AXIS2_PLACEMENT_3D('',#69555,#35378,#35379);
#32621=AXIS2_PLACEMENT_3D('',#69556,#35380,#35381);
#32622=AXIS2_PLACEMENT_3D('',#69565,#35386,#35387);
#32623=AXIS2_PLACEMENT_3D('',#69567,#35388,#35389);
#32624=AXIS2_PLACEMENT_3D('',#69569,#35391,#35392);
#32625=AXIS2_PLACEMENT_3D('',#69573,#35395,#35396);
#32626=AXIS2_PLACEMENT_3D('',#69574,#35397,#35398);
#32627=AXIS2_PLACEMENT_3D('',#69575,#35399,#35400);
#32628=AXIS2_PLACEMENT_3D('',#69584,#35405,#35406);
#32629=AXIS2_PLACEMENT_3D('',#69586,#35407,#35408);
#32630=AXIS2_PLACEMENT_3D('',#69588,#35410,#35411);
#32631=AXIS2_PLACEMENT_3D('',#69592,#35414,#35415);
#32632=AXIS2_PLACEMENT_3D('',#69593,#35416,#35417);
#32633=AXIS2_PLACEMENT_3D('',#69594,#35418,#35419);
#32634=AXIS2_PLACEMENT_3D('',#69603,#35424,#35425);
#32635=AXIS2_PLACEMENT_3D('',#69605,#35426,#35427);
#32636=AXIS2_PLACEMENT_3D('',#69607,#35429,#35430);
#32637=AXIS2_PLACEMENT_3D('',#69611,#35433,#35434);
#32638=AXIS2_PLACEMENT_3D('',#69612,#35435,#35436);
#32639=AXIS2_PLACEMENT_3D('',#69613,#35437,#35438);
#32640=AXIS2_PLACEMENT_3D('',#69622,#35443,#35444);
#32641=AXIS2_PLACEMENT_3D('',#69624,#35445,#35446);
#32642=AXIS2_PLACEMENT_3D('',#69626,#35448,#35449);
#32643=AXIS2_PLACEMENT_3D('',#69630,#35452,#35453);
#32644=AXIS2_PLACEMENT_3D('',#69631,#35454,#35455);
#32645=AXIS2_PLACEMENT_3D('',#69632,#35456,#35457);
#32646=AXIS2_PLACEMENT_3D('',#69641,#35462,#35463);
#32647=AXIS2_PLACEMENT_3D('',#69643,#35464,#35465);
#32648=AXIS2_PLACEMENT_3D('',#69645,#35467,#35468);
#32649=AXIS2_PLACEMENT_3D('',#69649,#35471,#35472);
#32650=AXIS2_PLACEMENT_3D('',#69650,#35473,#35474);
#32651=AXIS2_PLACEMENT_3D('',#69651,#35475,#35476);
#32652=AXIS2_PLACEMENT_3D('',#69660,#35481,#35482);
#32653=AXIS2_PLACEMENT_3D('',#69662,#35483,#35484);
#32654=AXIS2_PLACEMENT_3D('',#69664,#35486,#35487);
#32655=AXIS2_PLACEMENT_3D('',#69668,#35490,#35491);
#32656=AXIS2_PLACEMENT_3D('',#69669,#35492,#35493);
#32657=AXIS2_PLACEMENT_3D('',#69670,#35494,#35495);
#32658=AXIS2_PLACEMENT_3D('',#69679,#35500,#35501);
#32659=AXIS2_PLACEMENT_3D('',#69681,#35502,#35503);
#32660=AXIS2_PLACEMENT_3D('',#69683,#35505,#35506);
#32661=AXIS2_PLACEMENT_3D('',#69687,#35509,#35510);
#32662=AXIS2_PLACEMENT_3D('',#69688,#35511,#35512);
#32663=AXIS2_PLACEMENT_3D('',#69689,#35513,#35514);
#32664=AXIS2_PLACEMENT_3D('',#69698,#35519,#35520);
#32665=AXIS2_PLACEMENT_3D('',#69700,#35521,#35522);
#32666=AXIS2_PLACEMENT_3D('',#69702,#35524,#35525);
#32667=AXIS2_PLACEMENT_3D('',#69706,#35528,#35529);
#32668=AXIS2_PLACEMENT_3D('',#69707,#35530,#35531);
#32669=AXIS2_PLACEMENT_3D('',#69708,#35532,#35533);
#32670=AXIS2_PLACEMENT_3D('',#69717,#35538,#35539);
#32671=AXIS2_PLACEMENT_3D('',#69719,#35540,#35541);
#32672=AXIS2_PLACEMENT_3D('',#69721,#35543,#35544);
#32673=AXIS2_PLACEMENT_3D('',#69725,#35547,#35548);
#32674=AXIS2_PLACEMENT_3D('',#69726,#35549,#35550);
#32675=AXIS2_PLACEMENT_3D('',#69727,#35551,#35552);
#32676=AXIS2_PLACEMENT_3D('',#69736,#35557,#35558);
#32677=AXIS2_PLACEMENT_3D('',#69738,#35559,#35560);
#32678=AXIS2_PLACEMENT_3D('',#69740,#35562,#35563);
#32679=AXIS2_PLACEMENT_3D('',#69744,#35566,#35567);
#32680=AXIS2_PLACEMENT_3D('',#69745,#35568,#35569);
#32681=AXIS2_PLACEMENT_3D('',#69746,#35570,#35571);
#32682=AXIS2_PLACEMENT_3D('',#69755,#35576,#35577);
#32683=AXIS2_PLACEMENT_3D('',#69757,#35578,#35579);
#32684=AXIS2_PLACEMENT_3D('',#69759,#35581,#35582);
#32685=AXIS2_PLACEMENT_3D('',#69763,#35585,#35586);
#32686=AXIS2_PLACEMENT_3D('',#69764,#35587,#35588);
#32687=AXIS2_PLACEMENT_3D('',#69765,#35589,#35590);
#32688=AXIS2_PLACEMENT_3D('',#69774,#35595,#35596);
#32689=AXIS2_PLACEMENT_3D('',#69776,#35597,#35598);
#32690=AXIS2_PLACEMENT_3D('',#69778,#35600,#35601);
#32691=AXIS2_PLACEMENT_3D('',#69782,#35604,#35605);
#32692=AXIS2_PLACEMENT_3D('',#69783,#35606,#35607);
#32693=AXIS2_PLACEMENT_3D('',#69784,#35608,#35609);
#32694=AXIS2_PLACEMENT_3D('',#69793,#35614,#35615);
#32695=AXIS2_PLACEMENT_3D('',#69795,#35616,#35617);
#32696=AXIS2_PLACEMENT_3D('',#69797,#35619,#35620);
#32697=AXIS2_PLACEMENT_3D('',#69801,#35623,#35624);
#32698=AXIS2_PLACEMENT_3D('',#69802,#35625,#35626);
#32699=AXIS2_PLACEMENT_3D('',#69803,#35627,#35628);
#32700=AXIS2_PLACEMENT_3D('',#69812,#35633,#35634);
#32701=AXIS2_PLACEMENT_3D('',#69814,#35635,#35636);
#32702=AXIS2_PLACEMENT_3D('',#69816,#35638,#35639);
#32703=AXIS2_PLACEMENT_3D('',#69820,#35642,#35643);
#32704=AXIS2_PLACEMENT_3D('',#69821,#35644,#35645);
#32705=AXIS2_PLACEMENT_3D('',#69822,#35646,#35647);
#32706=AXIS2_PLACEMENT_3D('',#69831,#35652,#35653);
#32707=AXIS2_PLACEMENT_3D('',#69833,#35654,#35655);
#32708=AXIS2_PLACEMENT_3D('',#69835,#35657,#35658);
#32709=AXIS2_PLACEMENT_3D('',#69839,#35661,#35662);
#32710=AXIS2_PLACEMENT_3D('',#69840,#35663,#35664);
#32711=AXIS2_PLACEMENT_3D('',#69841,#35665,#35666);
#32712=AXIS2_PLACEMENT_3D('',#69850,#35671,#35672);
#32713=AXIS2_PLACEMENT_3D('',#69852,#35673,#35674);
#32714=AXIS2_PLACEMENT_3D('',#69854,#35676,#35677);
#32715=AXIS2_PLACEMENT_3D('',#69858,#35680,#35681);
#32716=AXIS2_PLACEMENT_3D('',#69859,#35682,#35683);
#32717=AXIS2_PLACEMENT_3D('',#69860,#35684,#35685);
#32718=AXIS2_PLACEMENT_3D('',#69869,#35690,#35691);
#32719=AXIS2_PLACEMENT_3D('',#69871,#35692,#35693);
#32720=AXIS2_PLACEMENT_3D('',#69873,#35695,#35696);
#32721=AXIS2_PLACEMENT_3D('',#69877,#35699,#35700);
#32722=AXIS2_PLACEMENT_3D('',#69878,#35701,#35702);
#32723=AXIS2_PLACEMENT_3D('',#69879,#35703,#35704);
#32724=AXIS2_PLACEMENT_3D('',#69888,#35709,#35710);
#32725=AXIS2_PLACEMENT_3D('',#69890,#35711,#35712);
#32726=AXIS2_PLACEMENT_3D('',#69892,#35714,#35715);
#32727=AXIS2_PLACEMENT_3D('',#69896,#35718,#35719);
#32728=AXIS2_PLACEMENT_3D('',#69897,#35720,#35721);
#32729=AXIS2_PLACEMENT_3D('',#69898,#35722,#35723);
#32730=AXIS2_PLACEMENT_3D('',#69904,#35727,#35728);
#32731=AXIS2_PLACEMENT_3D('',#69905,#35729,#35730);
#32732=AXIS2_PLACEMENT_3D('',#69906,#35731,#35732);
#32733=AXIS2_PLACEMENT_3D('',#69910,#35735,#35736);
#32734=AXIS2_PLACEMENT_3D('',#69911,#35737,#35738);
#32735=AXIS2_PLACEMENT_3D('',#69912,#35739,#35740);
#32736=AXIS2_PLACEMENT_3D('',#69913,#35741,#35742);
#32737=AXIS2_PLACEMENT_3D('',#69914,#35743,#35744);
#32738=AXIS2_PLACEMENT_3D('',#69915,#35745,#35746);
#32739=AXIS2_PLACEMENT_3D('',#69916,#35747,#35748);
#32740=AXIS2_PLACEMENT_3D('',#69918,#35749,#35750);
#32741=AXIS2_PLACEMENT_3D('',#69921,#35752,#35753);
#32742=AXIS2_PLACEMENT_3D('',#69922,#35754,#35755);
#32743=AXIS2_PLACEMENT_3D('',#69924,#35756,#35757);
#32744=AXIS2_PLACEMENT_3D('',#69925,#35758,#35759);
#32745=AXIS2_PLACEMENT_3D('',#69927,#35760,#35761);
#32746=AXIS2_PLACEMENT_3D('',#69929,#35763,#35764);
#32747=AXIS2_PLACEMENT_3D('',#69931,#35765,#35766);
#32748=AXIS2_PLACEMENT_3D('',#69934,#35769,#35770);
#32749=AXIS2_PLACEMENT_3D('',#69937,#35772,#35773);
#32750=AXIS2_PLACEMENT_3D('',#69938,#35774,#35775);
#32751=AXIS2_PLACEMENT_3D('',#69940,#35776,#35777);
#32752=AXIS2_PLACEMENT_3D('',#69941,#35778,#35779);
#32753=AXIS2_PLACEMENT_3D('',#69943,#35780,#35781);
#32754=AXIS2_PLACEMENT_3D('',#69945,#35783,#35784);
#32755=AXIS2_PLACEMENT_3D('',#69947,#35785,#35786);
#32756=AXIS2_PLACEMENT_3D('',#69948,#35787,#35788);
#34933=DIRECTION('axis',(0.,0.,1.));
#34934=DIRECTION('refdir',(1.,0.,0.));
#34935=DIRECTION('center_axis',(-1.,0.,0.));
#34936=DIRECTION('ref_axis',(0.,0.,-1.));
#34937=DIRECTION('center_axis',(-0.559437318248335,0.,0.828872660274852));
#34938=DIRECTION('ref_axis',(-0.828872660274852,0.,-0.559437318248335));
#34939=DIRECTION('center_axis',(-0.275920768781063,0.,-0.961180383359579));
#34940=DIRECTION('ref_axis',(0.961180383359579,0.,-0.275920768781063));
#34941=DIRECTION('center_axis',(-0.422885465331123,0.,0.906183139995266));
#34942=DIRECTION('ref_axis',(-0.906183139995266,0.,-0.422885465331123));
#34943=DIRECTION('center_axis',(-0.422885465331123,0.,-0.906183139995266));
#34944=DIRECTION('ref_axis',(0.906183139995266,0.,-0.422885465331123));
#34945=DIRECTION('center_axis',(-0.275920768781063,0.,0.961180383359579));
#34946=DIRECTION('ref_axis',(-0.961180383359579,0.,-0.275920768781063));
#34947=DIRECTION('center_axis',(-0.559437318248336,0.,-0.828872660274852));
#34948=DIRECTION('ref_axis',(0.828872660274852,0.,-0.559437318248336));
#34949=DIRECTION('center_axis',(-0.559437318248336,0.,-0.828872660274852));
#34950=DIRECTION('ref_axis',(0.828872660274852,0.,-0.559437318248336));
#34951=DIRECTION('center_axis',(-0.275920768781063,0.,0.961180383359579));
#34952=DIRECTION('ref_axis',(-0.961180383359579,0.,-0.275920768781063));
#34953=DIRECTION('center_axis',(-0.422885465331123,0.,-0.906183139995266));
#34954=DIRECTION('ref_axis',(0.906183139995266,0.,-0.422885465331123));
#34955=DIRECTION('center_axis',(-0.422885465331123,0.,0.906183139995266));
#34956=DIRECTION('ref_axis',(-0.906183139995266,0.,-0.422885465331123));
#34957=DIRECTION('center_axis',(-0.275920768781063,0.,-0.961180383359579));
#34958=DIRECTION('ref_axis',(0.961180383359579,0.,-0.275920768781063));
#34959=DIRECTION('center_axis',(-0.559437318248335,0.,0.828872660274852));
#34960=DIRECTION('ref_axis',(-0.828872660274852,0.,-0.559437318248335));
#34961=DIRECTION('',(-1.,0.,0.));
#34962=DIRECTION('center_axis',(-0.559437318248335,0.,0.828872660274852));
#34963=DIRECTION('ref_axis',(0.828872660274852,0.,0.559437318248335));
#34964=DIRECTION('',(0.,1.,0.));
#34965=DIRECTION('',(-0.828872660274852,0.,-0.559437318248335));
#34966=DIRECTION('',(0.,1.,0.));
#34967=DIRECTION('center_axis',(-0.275920768781063,0.,-0.961180383359579));
#34968=DIRECTION('ref_axis',(-0.961180383359579,0.,0.275920768781063));
#34969=DIRECTION('',(0.961180383359579,0.,-0.275920768781063));
#34970=DIRECTION('',(0.,-1.,0.));
#34971=DIRECTION('center_axis',(-0.559437318248336,0.,-0.828872660274852));
#34972=DIRECTION('ref_axis',(-0.828872660274852,0.,0.559437318248336));
#34973=DIRECTION('',(0.,1.,0.));
#34974=DIRECTION('',(0.828872660274852,0.,-0.559437318248336));
#34975=DIRECTION('',(0.,-1.,0.));
#34976=DIRECTION('center_axis',(-0.559437318248336,0.,-0.828872660274852));
#34977=DIRECTION('ref_axis',(-0.828872660274852,0.,0.559437318248336));
#34978=DIRECTION('',(0.,-1.,0.));
#34979=DIRECTION('',(-0.828872660274852,0.,0.559437318248336));
#34980=DIRECTION('',(0.,1.,0.));
#34981=DIRECTION('center_axis',(-0.275920768781063,0.,0.961180383359579));
#34982=DIRECTION('ref_axis',(0.961180383359579,0.,0.275920768781063));
#34983=DIRECTION('',(0.,1.,0.));
#34984=DIRECTION('',(-0.961180383359579,0.,-0.275920768781063));
#34985=DIRECTION('center_axis',(-0.275920768781063,0.,0.961180383359579));
#34986=DIRECTION('ref_axis',(0.961180383359579,0.,0.275920768781063));
#34987=DIRECTION('',(0.961180383359579,0.,0.275920768781063));
#34988=DIRECTION('',(0.,1.,0.));
#34989=DIRECTION('center_axis',(-0.422885465331123,0.,0.906183139995266));
#34990=DIRECTION('ref_axis',(0.906183139995266,0.,0.422885465331123));
#34991=DIRECTION('',(0.,1.,0.));
#34992=DIRECTION('',(-0.906183139995266,0.,-0.422885465331123));
#34993=DIRECTION('',(0.,1.,0.));
#34994=DIRECTION('center_axis',(-0.422885465331123,0.,0.906183139995266));
#34995=DIRECTION('ref_axis',(0.906183139995266,0.,0.422885465331123));
#34996=DIRECTION('',(0.,1.,0.));
#34997=DIRECTION('',(0.906183139995266,0.,0.422885465331123));
#34998=DIRECTION('',(0.,1.,0.));
#34999=DIRECTION('center_axis',(-0.422885465331123,0.,-0.906183139995266));
#35000=DIRECTION('ref_axis',(-0.906183139995266,0.,0.422885465331123));
#35001=DIRECTION('',(0.906183139995266,0.,-0.422885465331123));
#35002=DIRECTION('',(0.,-1.,0.));
#35003=DIRECTION('center_axis',(-0.422885465331123,0.,-0.906183139995266));
#35004=DIRECTION('ref_axis',(-0.906183139995266,0.,0.422885465331123));
#35005=DIRECTION('',(0.,-1.,0.));
#35006=DIRECTION('',(-0.906183139995266,0.,0.422885465331123));
#35007=DIRECTION('center_axis',(0.,1.,0.));
#35008=DIRECTION('ref_axis',(0.987688340595138,0.,-0.156434465040231));
#35009=DIRECTION('center_axis',(0.,-1.,0.));
#35010=DIRECTION('ref_axis',(1.,0.,0.));
#35011=DIRECTION('center_axis',(0.,1.,0.));
#35012=DIRECTION('ref_axis',(0.156434465040231,0.,0.987688340595138));
#35013=DIRECTION('center_axis',(0.,1.,0.));
#35014=DIRECTION('ref_axis',(1.,0.,0.));
#35015=DIRECTION('center_axis',(-0.682213967724262,0.,-0.731152584787826));
#35016=DIRECTION('ref_axis',(-0.731152584787826,0.,0.682213967724262));
#35017=DIRECTION('',(0.,-1.,0.));
#35018=DIRECTION('',(-0.731152584787826,0.,0.682213967724262));
#35019=DIRECTION('',(0.,1.,0.));
#35020=DIRECTION('',(0.731152584787826,0.,-0.682213967724262));
#35021=DIRECTION('center_axis',(0.,1.,0.));
#35022=DIRECTION('ref_axis',(0.951056516295153,0.,-0.309016994374948));
#35023=DIRECTION('center_axis',(0.,-1.,0.));
#35024=DIRECTION('ref_axis',(1.,0.,0.));
#35025=DIRECTION('',(-0.992510175710776,0.,-0.122161987175083));
#35026=DIRECTION('center_axis',(-0.122161987175083,0.,0.992510175710776));
#35027=DIRECTION('ref_axis',(0.992510175710776,0.,0.122161987175083));
#35028=DIRECTION('',(0.,1.,0.));
#35029=DIRECTION('',(0.992510175710776,0.,0.122161987175083));
#35030=DIRECTION('center_axis',(0.,1.,0.));
#35031=DIRECTION('ref_axis',(0.309016994374948,0.,0.951056516295153));
#35032=DIRECTION('center_axis',(0.,1.,0.));
#35033=DIRECTION('ref_axis',(1.,0.,0.));
#35034=DIRECTION('center_axis',(-0.788192245176467,0.,-0.615429106107016));
#35035=DIRECTION('ref_axis',(-0.615429106107016,0.,0.788192245176467));
#35036=DIRECTION('',(0.,-1.,0.));
#35037=DIRECTION('',(-0.615429106107016,0.,0.788192245176467));
#35038=DIRECTION('',(0.,1.,0.));
#35039=DIRECTION('',(0.615429106107016,0.,-0.788192245176467));
#35040=DIRECTION('center_axis',(0.,1.,0.));
#35041=DIRECTION('ref_axis',(0.891006524188368,0.,-0.453990499739547));
#35042=DIRECTION('center_axis',(0.,-1.,0.));
#35043=DIRECTION('ref_axis',(1.,0.,0.));
#35044=DIRECTION('',(-0.99940107358355,0.,0.0346048279875384));
#35045=DIRECTION('center_axis',(0.0346048279875384,0.,0.99940107358355));
#35046=DIRECTION('ref_axis',(0.99940107358355,0.,-0.0346048279875384));
#35047=DIRECTION('',(0.,1.,0.));
#35048=DIRECTION('',(0.99940107358355,0.,-0.0346048279875384));
#35049=DIRECTION('center_axis',(0.,1.,0.));
#35050=DIRECTION('ref_axis',(0.453990499739547,0.,0.891006524188368));
#35051=DIRECTION('center_axis',(0.,1.,0.));
#35052=DIRECTION('ref_axis',(1.,0.,0.));
#35053=DIRECTION('center_axis',(-0.874762613692339,0.,-0.484551720341748));
#35054=DIRECTION('ref_axis',(-0.484551720341748,0.,0.874762613692339));
#35055=DIRECTION('',(0.,-1.,0.));
#35056=DIRECTION('',(-0.484551720341748,0.,0.874762613692339));
#35057=DIRECTION('',(0.,1.,0.));
#35058=DIRECTION('',(0.484551720341748,0.,-0.874762613692339));
#35059=DIRECTION('center_axis',(0.,1.,0.));
#35060=DIRECTION('ref_axis',(0.809016994374947,0.,-0.587785252292473));
#35061=DIRECTION('center_axis',(0.,-1.,0.));
#35062=DIRECTION('ref_axis',(1.,0.,0.));
#35063=DIRECTION('',(-0.981683400202696,0.,0.190519557438267));
#35064=DIRECTION('center_axis',(0.190519557438267,0.,0.981683400202696));
#35065=DIRECTION('ref_axis',(0.981683400202696,0.,-0.190519557438267));
#35066=DIRECTION('',(0.,1.,0.));
#35067=DIRECTION('',(0.981683400202696,0.,-0.190519557438267));
#35068=DIRECTION('center_axis',(0.,1.,0.));
#35069=DIRECTION('ref_axis',(0.587785252292473,0.,0.809016994374947));
#35070=DIRECTION('center_axis',(0.,1.,0.));
#35071=DIRECTION('ref_axis',(1.,0.,0.));
#35072=DIRECTION('center_axis',(-0.939793423488437,0.,-0.341743063086705));
#35073=DIRECTION('ref_axis',(-0.341743063086705,0.,0.939793423488437));
#35074=DIRECTION('',(0.,-1.,0.));
#35075=DIRECTION('',(-0.341743063086705,0.,0.939793423488437));
#35076=DIRECTION('',(0.,1.,0.));
#35077=DIRECTION('',(0.341743063086705,0.,-0.939793423488437));
#35078=DIRECTION('center_axis',(0.,1.,0.));
#35079=DIRECTION('ref_axis',(0.707106781186547,0.,-0.707106781186548));
#35080=DIRECTION('center_axis',(0.,-1.,0.));
#35081=DIRECTION('ref_axis',(1.,0.,0.));
#35082=DIRECTION('',(-0.939793423488437,0.,0.341743063086706));
#35083=DIRECTION('center_axis',(0.341743063086706,0.,0.939793423488437));
#35084=DIRECTION('ref_axis',(0.939793423488437,0.,-0.341743063086706));
#35085=DIRECTION('',(0.,1.,0.));
#35086=DIRECTION('',(0.939793423488437,0.,-0.341743063086706));
#35087=DIRECTION('center_axis',(0.,1.,0.));
#35088=DIRECTION('ref_axis',(0.707106781186548,0.,0.707106781186547));
#35089=DIRECTION('center_axis',(0.,1.,0.));
#35090=DIRECTION('ref_axis',(1.,0.,0.));
#35091=DIRECTION('center_axis',(-0.981683400202696,0.,-0.190519557438267));
#35092=DIRECTION('ref_axis',(-0.190519557438267,0.,0.981683400202696));
#35093=DIRECTION('',(0.,-1.,0.));
#35094=DIRECTION('',(-0.190519557438267,0.,0.981683400202696));
#35095=DIRECTION('',(0.,1.,0.));
#35096=DIRECTION('',(0.190519557438267,0.,-0.981683400202696));
#35097=DIRECTION('center_axis',(0.,1.,0.));
#35098=DIRECTION('ref_axis',(0.587785252292473,0.,-0.809016994374948));
#35099=DIRECTION('center_axis',(0.,-1.,0.));
#35100=DIRECTION('ref_axis',(1.,0.,0.));
#35101=DIRECTION('',(-0.874762613692339,0.,0.484551720341749));
#35102=DIRECTION('center_axis',(0.484551720341749,0.,0.874762613692339));
#35103=DIRECTION('ref_axis',(0.874762613692339,0.,-0.484551720341749));
#35104=DIRECTION('',(0.,1.,0.));
#35105=DIRECTION('',(0.874762613692339,0.,-0.484551720341749));
#35106=DIRECTION('center_axis',(0.,1.,0.));
#35107=DIRECTION('ref_axis',(0.809016994374948,0.,0.587785252292473));
#35108=DIRECTION('center_axis',(0.,1.,0.));
#35109=DIRECTION('ref_axis',(1.,0.,0.));
#35110=DIRECTION('center_axis',(-0.99940107358355,0.,-0.0346048279875381));
#35111=DIRECTION('ref_axis',(-0.0346048279875381,0.,0.99940107358355));
#35112=DIRECTION('',(0.,-1.,0.));
#35113=DIRECTION('',(-0.0346048279875381,0.,0.99940107358355));
#35114=DIRECTION('',(0.,1.,0.));
#35115=DIRECTION('',(0.0346048279875381,0.,-0.99940107358355));
#35116=DIRECTION('center_axis',(0.,1.,0.));
#35117=DIRECTION('ref_axis',(0.453990499739547,0.,-0.891006524188368));
#35118=DIRECTION('center_axis',(0.,-1.,0.));
#35119=DIRECTION('ref_axis',(1.,0.,0.));
#35120=DIRECTION('',(-0.788192245176467,0.,0.615429106107016));
#35121=DIRECTION('center_axis',(0.615429106107016,0.,0.788192245176467));
#35122=DIRECTION('ref_axis',(0.788192245176467,0.,-0.615429106107016));
#35123=DIRECTION('',(0.,1.,0.));
#35124=DIRECTION('',(0.788192245176467,0.,-0.615429106107016));
#35125=DIRECTION('center_axis',(0.,1.,0.));
#35126=DIRECTION('ref_axis',(0.891006524188368,0.,0.453990499739547));
#35127=DIRECTION('center_axis',(0.,1.,0.));
#35128=DIRECTION('ref_axis',(1.,0.,0.));
#35129=DIRECTION('center_axis',(-0.992510175710776,0.,0.122161987175083));
#35130=DIRECTION('ref_axis',(0.122161987175083,0.,0.992510175710776));
#35131=DIRECTION('',(0.,-1.,0.));
#35132=DIRECTION('',(0.122161987175083,0.,0.992510175710776));
#35133=DIRECTION('',(0.,1.,0.));
#35134=DIRECTION('',(-0.122161987175083,0.,-0.992510175710776));
#35135=DIRECTION('center_axis',(0.,1.,0.));
#35136=DIRECTION('ref_axis',(0.309016994374947,0.,-0.951056516295154));
#35137=DIRECTION('center_axis',(0.,-1.,0.));
#35138=DIRECTION('ref_axis',(1.,0.,0.));
#35139=DIRECTION('',(-0.682213967724262,0.,0.731152584787827));
#35140=DIRECTION('center_axis',(0.731152584787827,0.,0.682213967724262));
#35141=DIRECTION('ref_axis',(0.682213967724262,0.,-0.731152584787827));
#35142=DIRECTION('',(0.,1.,0.));
#35143=DIRECTION('',(0.682213967724262,0.,-0.731152584787827));
#35144=DIRECTION('center_axis',(0.,1.,0.));
#35145=DIRECTION('ref_axis',(0.951056516295154,0.,0.309016994374947));
#35146=DIRECTION('center_axis',(0.,1.,0.));
#35147=DIRECTION('ref_axis',(1.,0.,0.));
#35148=DIRECTION('center_axis',(-0.961180383359579,0.,0.275920768781063));
#35149=DIRECTION('ref_axis',(0.275920768781063,0.,0.961180383359579));
#35150=DIRECTION('',(0.,-1.,0.));
#35151=DIRECTION('',(0.275920768781063,0.,0.961180383359579));
#35152=DIRECTION('',(0.,1.,0.));
#35153=DIRECTION('',(-0.275920768781063,0.,-0.961180383359579));
#35154=DIRECTION('center_axis',(0.,1.,0.));
#35155=DIRECTION('ref_axis',(0.156434465040231,0.,-0.987688340595138));
#35156=DIRECTION('center_axis',(0.,-1.,0.));
#35157=DIRECTION('ref_axis',(1.,0.,0.));
#35158=DIRECTION('',(-0.559437318248335,0.,0.828872660274852));
#35159=DIRECTION('center_axis',(0.828872660274853,0.,0.559437318248335));
#35160=DIRECTION('ref_axis',(0.559437318248335,0.,-0.828872660274853));
#35161=DIRECTION('',(0.,1.,0.));
#35162=DIRECTION('',(0.559437318248335,0.,-0.828872660274852));
#35163=DIRECTION('center_axis',(0.,1.,0.));
#35164=DIRECTION('ref_axis',(0.987688340595138,0.,0.156434465040231));
#35165=DIRECTION('center_axis',(0.,1.,0.));
#35166=DIRECTION('ref_axis',(1.,0.,0.));
#35167=DIRECTION('center_axis',(-0.906183139995266,0.,0.422885465331123));
#35168=DIRECTION('ref_axis',(0.422885465331123,0.,0.906183139995266));
#35169=DIRECTION('',(0.,-1.,0.));
#35170=DIRECTION('',(0.422885465331123,0.,0.906183139995266));
#35171=DIRECTION('',(0.,1.,0.));
#35172=DIRECTION('',(-0.422885465331123,0.,-0.906183139995266));
#35173=DIRECTION('center_axis',(0.,1.,0.));
#35174=DIRECTION('ref_axis',(-1.83697019872103E-16,0.,-1.));
#35175=DIRECTION('center_axis',(0.,-1.,0.));
#35176=DIRECTION('ref_axis',(1.,0.,0.));
#35177=DIRECTION('',(-0.422885465331123,0.,0.906183139995266));
#35178=DIRECTION('center_axis',(0.906183139995266,0.,0.422885465331123));
#35179=DIRECTION('ref_axis',(0.422885465331123,0.,-0.906183139995266));
#35180=DIRECTION('',(0.,1.,0.));
#35181=DIRECTION('',(0.422885465331123,0.,-0.906183139995266));
#35182=DIRECTION('center_axis',(0.,1.,0.));
#35183=DIRECTION('ref_axis',(1.,0.,-1.83697019872103E-16));
#35184=DIRECTION('center_axis',(0.,1.,0.));
#35185=DIRECTION('ref_axis',(1.,0.,0.));
#35186=DIRECTION('center_axis',(-0.828872660274852,0.,0.559437318248335));
#35187=DIRECTION('ref_axis',(0.559437318248335,0.,0.828872660274853));
#35188=DIRECTION('',(0.,-1.,0.));
#35189=DIRECTION('',(0.559437318248335,0.,0.828872660274852));
#35190=DIRECTION('',(0.,1.,0.));
#35191=DIRECTION('',(-0.559437318248335,0.,-0.828872660274852));
#35192=DIRECTION('center_axis',(0.,1.,0.));
#35193=DIRECTION('ref_axis',(-0.156434465040231,0.,-0.987688340595138));
#35194=DIRECTION('center_axis',(0.,-1.,0.));
#35195=DIRECTION('ref_axis',(1.,0.,0.));
#35196=DIRECTION('',(-0.275920768781063,0.,0.961180383359579));
#35197=DIRECTION('center_axis',(0.961180383359579,0.,0.275920768781063));
#35198=DIRECTION('ref_axis',(0.275920768781063,0.,-0.961180383359579));
#35199=DIRECTION('',(0.,1.,0.));
#35200=DIRECTION('',(0.275920768781063,0.,-0.961180383359579));
#35201=DIRECTION('center_axis',(0.,1.,0.));
#35202=DIRECTION('ref_axis',(0.987688340595138,0.,-0.156434465040231));
#35203=DIRECTION('center_axis',(0.,1.,0.));
#35204=DIRECTION('ref_axis',(1.,0.,0.));
#35205=DIRECTION('center_axis',(-0.731152584787826,0.,0.682213967724262));
#35206=DIRECTION('ref_axis',(0.682213967724262,0.,0.731152584787826));
#35207=DIRECTION('',(0.,-1.,0.));
#35208=DIRECTION('',(0.682213967724262,0.,0.731152584787826));
#35209=DIRECTION('',(0.,1.,0.));
#35210=DIRECTION('',(-0.682213967724262,0.,-0.731152584787826));
#35211=DIRECTION('center_axis',(0.,1.,0.));
#35212=DIRECTION('ref_axis',(-0.309016994374948,0.,-0.951056516295153));
#35213=DIRECTION('center_axis',(0.,-1.,0.));
#35214=DIRECTION('ref_axis',(1.,0.,0.));
#35215=DIRECTION('',(-0.122161987175083,0.,0.992510175710776));
#35216=DIRECTION('center_axis',(0.992510175710776,0.,0.122161987175083));
#35217=DIRECTION('ref_axis',(0.122161987175083,0.,-0.992510175710776));
#35218=DIRECTION('',(0.,1.,0.));
#35219=DIRECTION('',(0.122161987175083,0.,-0.992510175710776));
#35220=DIRECTION('center_axis',(0.,1.,0.));
#35221=DIRECTION('ref_axis',(0.951056516295153,0.,-0.309016994374948));
#35222=DIRECTION('center_axis',(0.,1.,0.));
#35223=DIRECTION('ref_axis',(1.,0.,0.));
#35224=DIRECTION('center_axis',(-0.615429106107016,0.,0.788192245176467));
#35225=DIRECTION('ref_axis',(0.788192245176467,0.,0.615429106107016));
#35226=DIRECTION('',(0.,-1.,0.));
#35227=DIRECTION('',(0.788192245176467,0.,0.615429106107016));
#35228=DIRECTION('',(0.,1.,0.));
#35229=DIRECTION('',(-0.788192245176467,0.,-0.615429106107016));
#35230=DIRECTION('center_axis',(0.,1.,0.));
#35231=DIRECTION('ref_axis',(-0.453990499739547,0.,-0.891006524188368));
#35232=DIRECTION('center_axis',(0.,-1.,0.));
#35233=DIRECTION('ref_axis',(1.,0.,0.));
#35234=DIRECTION('',(0.0346048279875384,0.,0.99940107358355));
#35235=DIRECTION('center_axis',(0.99940107358355,0.,-0.0346048279875384));
#35236=DIRECTION('ref_axis',(-0.0346048279875384,0.,-0.99940107358355));
#35237=DIRECTION('',(0.,1.,0.));
#35238=DIRECTION('',(-0.0346048279875384,0.,-0.99940107358355));
#35239=DIRECTION('center_axis',(0.,1.,0.));
#35240=DIRECTION('ref_axis',(0.891006524188368,0.,-0.453990499739547));
#35241=DIRECTION('center_axis',(0.,1.,0.));
#35242=DIRECTION('ref_axis',(1.,0.,0.));
#35243=DIRECTION('center_axis',(-0.484551720341748,0.,0.874762613692339));
#35244=DIRECTION('ref_axis',(0.874762613692339,0.,0.484551720341748));
#35245=DIRECTION('',(0.,-1.,0.));
#35246=DIRECTION('',(0.874762613692339,0.,0.484551720341748));
#35247=DIRECTION('',(0.,1.,0.));
#35248=DIRECTION('',(-0.874762613692339,0.,-0.484551720341748));
#35249=DIRECTION('center_axis',(0.,1.,0.));
#35250=DIRECTION('ref_axis',(-0.587785252292473,0.,-0.809016994374947));
#35251=DIRECTION('center_axis',(0.,-1.,0.));
#35252=DIRECTION('ref_axis',(1.,0.,0.));
#35253=DIRECTION('',(0.190519557438267,0.,0.981683400202696));
#35254=DIRECTION('center_axis',(0.981683400202696,0.,-0.190519557438267));
#35255=DIRECTION('ref_axis',(-0.190519557438267,0.,-0.981683400202696));
#35256=DIRECTION('',(0.,1.,0.));
#35257=DIRECTION('',(-0.190519557438267,0.,-0.981683400202696));
#35258=DIRECTION('center_axis',(0.,1.,0.));
#35259=DIRECTION('ref_axis',(0.809016994374947,0.,-0.587785252292473));
#35260=DIRECTION('center_axis',(0.,1.,0.));
#35261=DIRECTION('ref_axis',(1.,0.,0.));
#35262=DIRECTION('center_axis',(-0.341743063086705,0.,0.939793423488437));
#35263=DIRECTION('ref_axis',(0.939793423488437,0.,0.341743063086705));
#35264=DIRECTION('',(0.,-1.,0.));
#35265=DIRECTION('',(0.939793423488437,0.,0.341743063086705));
#35266=DIRECTION('',(0.,1.,0.));
#35267=DIRECTION('',(-0.939793423488437,0.,-0.341743063086705));
#35268=DIRECTION('center_axis',(0.,1.,0.));
#35269=DIRECTION('ref_axis',(-0.707106781186548,0.,-0.707106781186547));
#35270=DIRECTION('center_axis',(0.,-1.,0.));
#35271=DIRECTION('ref_axis',(1.,0.,0.));
#35272=DIRECTION('',(0.341743063086706,0.,0.939793423488437));
#35273=DIRECTION('center_axis',(0.939793423488437,0.,-0.341743063086706));
#35274=DIRECTION('ref_axis',(-0.341743063086706,0.,-0.939793423488437));
#35275=DIRECTION('',(0.,1.,0.));
#35276=DIRECTION('',(-0.341743063086706,0.,-0.939793423488437));
#35277=DIRECTION('center_axis',(0.,1.,0.));
#35278=DIRECTION('ref_axis',(0.707106781186547,0.,-0.707106781186548));
#35279=DIRECTION('center_axis',(0.,1.,0.));
#35280=DIRECTION('ref_axis',(1.,0.,0.));
#35281=DIRECTION('center_axis',(-0.190519557438267,0.,0.981683400202696));
#35282=DIRECTION('ref_axis',(0.981683400202696,0.,0.190519557438267));
#35283=DIRECTION('',(0.,-1.,0.));
#35284=DIRECTION('',(0.981683400202696,0.,0.190519557438267));
#35285=DIRECTION('',(0.,1.,0.));
#35286=DIRECTION('',(-0.981683400202696,0.,-0.190519557438267));
#35287=DIRECTION('center_axis',(0.,1.,0.));
#35288=DIRECTION('ref_axis',(-0.809016994374947,0.,-0.587785252292473));
#35289=DIRECTION('center_axis',(0.,-1.,0.));
#35290=DIRECTION('ref_axis',(1.,0.,0.));
#35291=DIRECTION('',(0.484551720341748,0.,0.874762613692339));
#35292=DIRECTION('center_axis',(0.874762613692339,0.,-0.484551720341748));
#35293=DIRECTION('ref_axis',(-0.484551720341748,0.,-0.874762613692339));
#35294=DIRECTION('',(0.,1.,0.));
#35295=DIRECTION('',(-0.484551720341748,0.,-0.874762613692339));
#35296=DIRECTION('center_axis',(0.,1.,0.));
#35297=DIRECTION('ref_axis',(0.587785252292473,0.,-0.809016994374947));
#35298=DIRECTION('center_axis',(0.,1.,0.));
#35299=DIRECTION('ref_axis',(1.,0.,0.));
#35300=DIRECTION('center_axis',(-0.0346048279875381,0.,0.99940107358355));
#35301=DIRECTION('ref_axis',(0.99940107358355,0.,0.0346048279875381));
#35302=DIRECTION('',(0.,-1.,0.));
#35303=DIRECTION('',(0.99940107358355,0.,0.0346048279875381));
#35304=DIRECTION('',(0.,1.,0.));
#35305=DIRECTION('',(-0.99940107358355,0.,-0.0346048279875381));
#35306=DIRECTION('center_axis',(0.,1.,0.));
#35307=DIRECTION('ref_axis',(-0.891006524188368,0.,-0.453990499739547));
#35308=DIRECTION('center_axis',(0.,-1.,0.));
#35309=DIRECTION('ref_axis',(1.,0.,0.));
#35310=DIRECTION('',(0.615429106107016,0.,0.788192245176467));
#35311=DIRECTION('center_axis',(0.788192245176467,0.,-0.615429106107016));
#35312=DIRECTION('ref_axis',(-0.615429106107016,0.,-0.788192245176467));
#35313=DIRECTION('',(0.,1.,0.));
#35314=DIRECTION('',(-0.615429106107016,0.,-0.788192245176467));
#35315=DIRECTION('center_axis',(0.,1.,0.));
#35316=DIRECTION('ref_axis',(0.453990499739547,0.,-0.891006524188368));
#35317=DIRECTION('center_axis',(0.,1.,0.));
#35318=DIRECTION('ref_axis',(1.,0.,0.));
#35319=DIRECTION('center_axis',(0.122161987175083,0.,0.992510175710776));
#35320=DIRECTION('ref_axis',(0.992510175710776,0.,-0.122161987175083));
#35321=DIRECTION('',(0.,-1.,0.));
#35322=DIRECTION('',(0.992510175710776,0.,-0.122161987175083));
#35323=DIRECTION('',(0.,1.,0.));
#35324=DIRECTION('',(-0.992510175710776,0.,0.122161987175083));
#35325=DIRECTION('center_axis',(0.,1.,0.));
#35326=DIRECTION('ref_axis',(-0.951056516295154,0.,-0.309016994374947));
#35327=DIRECTION('center_axis',(0.,-1.,0.));
#35328=DIRECTION('ref_axis',(1.,0.,0.));
#35329=DIRECTION('',(0.731152584787827,0.,0.682213967724262));
#35330=DIRECTION('center_axis',(0.682213967724262,0.,-0.731152584787827));
#35331=DIRECTION('ref_axis',(-0.731152584787827,0.,-0.682213967724262));
#35332=DIRECTION('',(0.,1.,0.));
#35333=DIRECTION('',(-0.731152584787827,0.,-0.682213967724262));
#35334=DIRECTION('center_axis',(0.,1.,0.));
#35335=DIRECTION('ref_axis',(0.309016994374947,0.,-0.951056516295154));
#35336=DIRECTION('center_axis',(0.,1.,0.));
#35337=DIRECTION('ref_axis',(1.,0.,0.));
#35338=DIRECTION('center_axis',(0.275920768781063,0.,0.961180383359579));
#35339=DIRECTION('ref_axis',(0.961180383359579,0.,-0.275920768781063));
#35340=DIRECTION('',(0.,-1.,0.));
#35341=DIRECTION('',(0.961180383359579,0.,-0.275920768781063));
#35342=DIRECTION('',(0.,1.,0.));
#35343=DIRECTION('',(-0.961180383359579,0.,0.275920768781063));
#35344=DIRECTION('center_axis',(0.,1.,0.));
#35345=DIRECTION('ref_axis',(-0.987688340595138,0.,-0.156434465040231));
#35346=DIRECTION('center_axis',(0.,-1.,0.));
#35347=DIRECTION('ref_axis',(1.,0.,0.));
#35348=DIRECTION('',(0.828872660274852,0.,0.559437318248335));
#35349=DIRECTION('center_axis',(0.559437318248335,0.,-0.828872660274853));
#35350=DIRECTION('ref_axis',(-0.828872660274853,0.,-0.559437318248335));
#35351=DIRECTION('',(0.,1.,0.));
#35352=DIRECTION('',(-0.828872660274852,0.,-0.559437318248335));
#35353=DIRECTION('center_axis',(0.,1.,0.));
#35354=DIRECTION('ref_axis',(0.156434465040231,0.,-0.987688340595138));
#35355=DIRECTION('center_axis',(0.,1.,0.));
#35356=DIRECTION('ref_axis',(1.,0.,0.));
#35357=DIRECTION('center_axis',(0.422885465331123,0.,0.906183139995266));
#35358=DIRECTION('ref_axis',(0.906183139995266,0.,-0.422885465331123));
#35359=DIRECTION('',(0.,-1.,0.));
#35360=DIRECTION('',(0.906183139995266,0.,-0.422885465331123));
#35361=DIRECTION('',(0.,1.,0.));
#35362=DIRECTION('',(-0.906183139995266,0.,0.422885465331123));
#35363=DIRECTION('center_axis',(0.,1.,0.));
#35364=DIRECTION('ref_axis',(-1.,0.,1.22464679914735E-16));
#35365=DIRECTION('center_axis',(0.,-1.,0.));
#35366=DIRECTION('ref_axis',(1.,0.,0.));
#35367=DIRECTION('',(0.906183139995266,0.,0.422885465331123));
#35368=DIRECTION('center_axis',(0.,-1.,0.));
#35369=DIRECTION('ref_axis',(1.,0.,0.));
#35370=DIRECTION('center_axis',(0.422885465331123,0.,-0.906183139995266));
#35371=DIRECTION('ref_axis',(-0.906183139995266,0.,-0.422885465331123));
#35372=DIRECTION('',(0.,1.,0.));
#35373=DIRECTION('',(-0.906183139995266,0.,-0.422885465331123));
#35374=DIRECTION('center_axis',(0.,1.,0.));
#35375=DIRECTION('ref_axis',(-1.22464679914735E-16,0.,-1.));
#35376=DIRECTION('center_axis',(0.,1.,0.));
#35377=DIRECTION('ref_axis',(1.,0.,0.));
#35378=DIRECTION('center_axis',(0.,1.,0.));
#35379=DIRECTION('ref_axis',(1.,0.,0.));
#35380=DIRECTION('center_axis',(0.559437318248335,0.,0.828872660274852));
#35381=DIRECTION('ref_axis',(0.828872660274852,0.,-0.559437318248335));
#35382=DIRECTION('',(0.,-1.,0.));
#35383=DIRECTION('',(0.828872660274852,0.,-0.559437318248335));
#35384=DIRECTION('',(0.,1.,0.));
#35385=DIRECTION('',(-0.828872660274852,0.,0.559437318248335));
#35386=DIRECTION('center_axis',(0.,1.,0.));
#35387=DIRECTION('ref_axis',(-0.987688340595138,0.,0.156434465040231));
#35388=DIRECTION('center_axis',(0.,-1.,0.));
#35389=DIRECTION('ref_axis',(1.,0.,0.));
#35390=DIRECTION('',(0.961180383359579,0.,0.275920768781063));
#35391=DIRECTION('center_axis',(0.275920768781063,0.,-0.961180383359579));
#35392=DIRECTION('ref_axis',(-0.961180383359579,0.,-0.275920768781063));
#35393=DIRECTION('',(0.,1.,0.));
#35394=DIRECTION('',(-0.961180383359579,0.,-0.275920768781063));
#35395=DIRECTION('center_axis',(0.,1.,0.));
#35396=DIRECTION('ref_axis',(-0.156434465040231,0.,-0.987688340595138));
#35397=DIRECTION('center_axis',(0.,1.,0.));
#35398=DIRECTION('ref_axis',(1.,0.,0.));
#35399=DIRECTION('center_axis',(0.682213967724262,0.,0.731152584787826));
#35400=DIRECTION('ref_axis',(0.731152584787826,0.,-0.682213967724262));
#35401=DIRECTION('',(0.,-1.,0.));
#35402=DIRECTION('',(0.731152584787826,0.,-0.682213967724262));
#35403=DIRECTION('',(0.,1.,0.));
#35404=DIRECTION('',(-0.731152584787826,0.,0.682213967724262));
#35405=DIRECTION('center_axis',(0.,1.,0.));
#35406=DIRECTION('ref_axis',(-0.951056516295153,0.,0.309016994374948));
#35407=DIRECTION('center_axis',(0.,-1.,0.));
#35408=DIRECTION('ref_axis',(1.,0.,0.));
#35409=DIRECTION('',(0.992510175710776,0.,0.122161987175083));
#35410=DIRECTION('center_axis',(0.122161987175083,0.,-0.992510175710776));
#35411=DIRECTION('ref_axis',(-0.992510175710776,0.,-0.122161987175083));
#35412=DIRECTION('',(0.,1.,0.));
#35413=DIRECTION('',(-0.992510175710776,0.,-0.122161987175083));
#35414=DIRECTION('center_axis',(0.,1.,0.));
#35415=DIRECTION('ref_axis',(-0.309016994374948,0.,-0.951056516295153));
#35416=DIRECTION('center_axis',(0.,1.,0.));
#35417=DIRECTION('ref_axis',(1.,0.,0.));
#35418=DIRECTION('center_axis',(0.788192245176467,0.,0.615429106107016));
#35419=DIRECTION('ref_axis',(0.615429106107016,0.,-0.788192245176467));
#35420=DIRECTION('',(0.,-1.,0.));
#35421=DIRECTION('',(0.615429106107016,0.,-0.788192245176467));
#35422=DIRECTION('',(0.,1.,0.));
#35423=DIRECTION('',(-0.615429106107016,0.,0.788192245176467));
#35424=DIRECTION('center_axis',(0.,1.,0.));
#35425=DIRECTION('ref_axis',(-0.891006524188368,0.,0.453990499739547));
#35426=DIRECTION('center_axis',(0.,-1.,0.));
#35427=DIRECTION('ref_axis',(1.,0.,0.));
#35428=DIRECTION('',(0.99940107358355,0.,-0.0346048279875384));
#35429=DIRECTION('center_axis',(-0.0346048279875384,0.,-0.99940107358355));
#35430=DIRECTION('ref_axis',(-0.99940107358355,0.,0.0346048279875384));
#35431=DIRECTION('',(0.,1.,0.));
#35432=DIRECTION('',(-0.99940107358355,0.,0.0346048279875384));
#35433=DIRECTION('center_axis',(0.,1.,0.));
#35434=DIRECTION('ref_axis',(-0.453990499739547,0.,-0.891006524188368));
#35435=DIRECTION('center_axis',(0.,1.,0.));
#35436=DIRECTION('ref_axis',(1.,0.,0.));
#35437=DIRECTION('center_axis',(0.874762613692339,0.,0.484551720341748));
#35438=DIRECTION('ref_axis',(0.484551720341748,0.,-0.874762613692339));
#35439=DIRECTION('',(0.,-1.,0.));
#35440=DIRECTION('',(0.484551720341748,0.,-0.874762613692339));
#35441=DIRECTION('',(0.,1.,0.));
#35442=DIRECTION('',(-0.484551720341748,0.,0.874762613692339));
#35443=DIRECTION('center_axis',(0.,1.,0.));
#35444=DIRECTION('ref_axis',(-0.809016994374947,0.,0.587785252292473));
#35445=DIRECTION('center_axis',(0.,-1.,0.));
#35446=DIRECTION('ref_axis',(1.,0.,0.));
#35447=DIRECTION('',(0.981683400202696,0.,-0.190519557438267));
#35448=DIRECTION('center_axis',(-0.190519557438267,0.,-0.981683400202696));
#35449=DIRECTION('ref_axis',(-0.981683400202696,0.,0.190519557438267));
#35450=DIRECTION('',(0.,1.,0.));
#35451=DIRECTION('',(-0.981683400202696,0.,0.190519557438267));
#35452=DIRECTION('center_axis',(0.,1.,0.));
#35453=DIRECTION('ref_axis',(-0.587785252292473,0.,-0.809016994374947));
#35454=DIRECTION('center_axis',(0.,1.,0.));
#35455=DIRECTION('ref_axis',(1.,0.,0.));
#35456=DIRECTION('center_axis',(0.939793423488437,0.,0.341743063086706));
#35457=DIRECTION('ref_axis',(0.341743063086706,0.,-0.939793423488437));
#35458=DIRECTION('',(0.,-1.,0.));
#35459=DIRECTION('',(0.341743063086706,0.,-0.939793423488437));
#35460=DIRECTION('',(0.,1.,0.));
#35461=DIRECTION('',(-0.341743063086706,0.,0.939793423488437));
#35462=DIRECTION('center_axis',(0.,1.,0.));
#35463=DIRECTION('ref_axis',(-0.707106781186547,0.,0.707106781186548));
#35464=DIRECTION('center_axis',(0.,-1.,0.));
#35465=DIRECTION('ref_axis',(1.,0.,0.));
#35466=DIRECTION('',(0.939793423488437,0.,-0.341743063086706));
#35467=DIRECTION('center_axis',(-0.341743063086706,0.,-0.939793423488437));
#35468=DIRECTION('ref_axis',(-0.939793423488437,0.,0.341743063086706));
#35469=DIRECTION('',(0.,1.,0.));
#35470=DIRECTION('',(-0.939793423488437,0.,0.341743063086706));
#35471=DIRECTION('center_axis',(0.,1.,0.));
#35472=DIRECTION('ref_axis',(-0.707106781186548,0.,-0.707106781186547));
#35473=DIRECTION('center_axis',(0.,1.,0.));
#35474=DIRECTION('ref_axis',(1.,0.,0.));
#35475=DIRECTION('center_axis',(0.981683400202696,0.,0.190519557438267));
#35476=DIRECTION('ref_axis',(0.190519557438267,0.,-0.981683400202696));
#35477=DIRECTION('',(0.,-1.,0.));
#35478=DIRECTION('',(0.190519557438267,0.,-0.981683400202696));
#35479=DIRECTION('',(0.,1.,0.));
#35480=DIRECTION('',(-0.190519557438267,0.,0.981683400202696));
#35481=DIRECTION('center_axis',(0.,1.,0.));
#35482=DIRECTION('ref_axis',(-0.587785252292473,0.,0.809016994374947));
#35483=DIRECTION('center_axis',(0.,-1.,0.));
#35484=DIRECTION('ref_axis',(1.,0.,0.));
#35485=DIRECTION('',(0.874762613692339,0.,-0.484551720341748));
#35486=DIRECTION('center_axis',(-0.484551720341748,0.,-0.874762613692339));
#35487=DIRECTION('ref_axis',(-0.874762613692339,0.,0.484551720341748));
#35488=DIRECTION('',(0.,1.,0.));
#35489=DIRECTION('',(-0.874762613692339,0.,0.484551720341748));
#35490=DIRECTION('center_axis',(0.,1.,0.));
#35491=DIRECTION('ref_axis',(-0.809016994374947,0.,-0.587785252292473));
#35492=DIRECTION('center_axis',(0.,1.,0.));
#35493=DIRECTION('ref_axis',(1.,0.,0.));
#35494=DIRECTION('center_axis',(0.99940107358355,0.,0.0346048279875382));
#35495=DIRECTION('ref_axis',(0.0346048279875382,0.,-0.99940107358355));
#35496=DIRECTION('',(0.,-1.,0.));
#35497=DIRECTION('',(0.0346048279875382,0.,-0.99940107358355));
#35498=DIRECTION('',(0.,1.,0.));
#35499=DIRECTION('',(-0.0346048279875382,0.,0.99940107358355));
#35500=DIRECTION('center_axis',(0.,1.,0.));
#35501=DIRECTION('ref_axis',(-0.453990499739547,0.,0.891006524188368));
#35502=DIRECTION('center_axis',(0.,-1.,0.));
#35503=DIRECTION('ref_axis',(1.,0.,0.));
#35504=DIRECTION('',(0.788192245176467,0.,-0.615429106107016));
#35505=DIRECTION('center_axis',(-0.615429106107016,0.,-0.788192245176467));
#35506=DIRECTION('ref_axis',(-0.788192245176467,0.,0.615429106107016));
#35507=DIRECTION('',(0.,1.,0.));
#35508=DIRECTION('',(-0.788192245176467,0.,0.615429106107016));
#35509=DIRECTION('center_axis',(0.,1.,0.));
#35510=DIRECTION('ref_axis',(-0.891006524188368,0.,-0.453990499739547));
#35511=DIRECTION('center_axis',(0.,1.,0.));
#35512=DIRECTION('ref_axis',(1.,0.,0.));
#35513=DIRECTION('center_axis',(0.992510175710776,0.,-0.122161987175083));
#35514=DIRECTION('ref_axis',(-0.122161987175083,0.,-0.992510175710776));
#35515=DIRECTION('',(0.,-1.,0.));
#35516=DIRECTION('',(-0.122161987175083,0.,-0.992510175710776));
#35517=DIRECTION('',(0.,1.,0.));
#35518=DIRECTION('',(0.122161987175083,0.,0.992510175710776));
#35519=DIRECTION('center_axis',(0.,1.,0.));
#35520=DIRECTION('ref_axis',(-0.309016994374947,0.,0.951056516295154));
#35521=DIRECTION('center_axis',(0.,-1.,0.));
#35522=DIRECTION('ref_axis',(1.,0.,0.));
#35523=DIRECTION('',(0.682213967724262,0.,-0.731152584787827));
#35524=DIRECTION('center_axis',(-0.731152584787827,0.,-0.682213967724262));
#35525=DIRECTION('ref_axis',(-0.682213967724262,0.,0.731152584787827));
#35526=DIRECTION('',(0.,1.,0.));
#35527=DIRECTION('',(-0.682213967724262,0.,0.731152584787827));
#35528=DIRECTION('center_axis',(0.,1.,0.));
#35529=DIRECTION('ref_axis',(-0.951056516295154,0.,-0.309016994374947));
#35530=DIRECTION('center_axis',(0.,1.,0.));
#35531=DIRECTION('ref_axis',(1.,0.,0.));
#35532=DIRECTION('center_axis',(0.961180383359579,0.,-0.275920768781063));
#35533=DIRECTION('ref_axis',(-0.275920768781063,0.,-0.961180383359579));
#35534=DIRECTION('',(0.,-1.,0.));
#35535=DIRECTION('',(-0.275920768781063,0.,-0.961180383359579));
#35536=DIRECTION('',(0.,1.,0.));
#35537=DIRECTION('',(0.275920768781063,0.,0.961180383359579));
#35538=DIRECTION('center_axis',(0.,1.,0.));
#35539=DIRECTION('ref_axis',(-0.156434465040231,0.,0.987688340595138));
#35540=DIRECTION('center_axis',(0.,-1.,0.));
#35541=DIRECTION('ref_axis',(1.,0.,0.));
#35542=DIRECTION('',(0.559437318248335,0.,-0.828872660274852));
#35543=DIRECTION('center_axis',(-0.828872660274852,0.,-0.559437318248335));
#35544=DIRECTION('ref_axis',(-0.559437318248335,0.,0.828872660274853));
#35545=DIRECTION('',(0.,1.,0.));
#35546=DIRECTION('',(-0.559437318248335,0.,0.828872660274852));
#35547=DIRECTION('center_axis',(0.,1.,0.));
#35548=DIRECTION('ref_axis',(-0.987688340595138,0.,-0.156434465040231));
#35549=DIRECTION('center_axis',(0.,1.,0.));
#35550=DIRECTION('ref_axis',(1.,0.,0.));
#35551=DIRECTION('center_axis',(0.906183139995266,0.,-0.422885465331123));
#35552=DIRECTION('ref_axis',(-0.422885465331123,0.,-0.906183139995266));
#35553=DIRECTION('',(0.,-1.,0.));
#35554=DIRECTION('',(-0.422885465331123,0.,-0.906183139995266));
#35555=DIRECTION('',(0.,1.,0.));
#35556=DIRECTION('',(0.422885465331123,0.,0.906183139995266));
#35557=DIRECTION('center_axis',(0.,1.,0.));
#35558=DIRECTION('ref_axis',(6.12323399573677E-17,0.,1.));
#35559=DIRECTION('center_axis',(0.,-1.,0.));
#35560=DIRECTION('ref_axis',(1.,0.,0.));
#35561=DIRECTION('',(0.422885465331123,0.,-0.906183139995266));
#35562=DIRECTION('center_axis',(-0.906183139995266,0.,-0.422885465331123));
#35563=DIRECTION('ref_axis',(-0.422885465331123,0.,0.906183139995266));
#35564=DIRECTION('',(0.,1.,0.));
#35565=DIRECTION('',(-0.422885465331123,0.,0.906183139995266));
#35566=DIRECTION('center_axis',(0.,1.,0.));
#35567=DIRECTION('ref_axis',(-1.,0.,6.12323399573677E-17));
#35568=DIRECTION('center_axis',(0.,1.,0.));
#35569=DIRECTION('ref_axis',(1.,0.,0.));
#35570=DIRECTION('center_axis',(0.828872660274852,0.,-0.559437318248335));
#35571=DIRECTION('ref_axis',(-0.559437318248335,0.,-0.828872660274853));
#35572=DIRECTION('',(0.,-1.,0.));
#35573=DIRECTION('',(-0.559437318248335,0.,-0.828872660274852));
#35574=DIRECTION('',(0.,1.,0.));
#35575=DIRECTION('',(0.559437318248335,0.,0.828872660274852));
#35576=DIRECTION('center_axis',(0.,1.,0.));
#35577=DIRECTION('ref_axis',(0.156434465040231,0.,0.987688340595138));
#35578=DIRECTION('center_axis',(0.,-1.,0.));
#35579=DIRECTION('ref_axis',(1.,0.,0.));
#35580=DIRECTION('',(0.275920768781063,0.,-0.961180383359579));
#35581=DIRECTION('center_axis',(-0.961180383359579,0.,-0.275920768781063));
#35582=DIRECTION('ref_axis',(-0.275920768781063,0.,0.961180383359579));
#35583=DIRECTION('',(0.,1.,0.));
#35584=DIRECTION('',(-0.275920768781063,0.,0.961180383359579));
#35585=DIRECTION('center_axis',(0.,1.,0.));
#35586=DIRECTION('ref_axis',(-0.987688340595138,0.,0.156434465040231));
#35587=DIRECTION('center_axis',(0.,1.,0.));
#35588=DIRECTION('ref_axis',(1.,0.,0.));
#35589=DIRECTION('center_axis',(0.731152584787827,0.,-0.682213967724262));
#35590=DIRECTION('ref_axis',(-0.682213967724262,0.,-0.731152584787827));
#35591=DIRECTION('',(0.,-1.,0.));
#35592=DIRECTION('',(-0.682213967724262,0.,-0.731152584787826));
#35593=DIRECTION('',(0.,1.,0.));
#35594=DIRECTION('',(0.682213967724262,0.,0.731152584787826));
#35595=DIRECTION('center_axis',(0.,1.,0.));
#35596=DIRECTION('ref_axis',(0.309016994374948,0.,0.951056516295154));
#35597=DIRECTION('center_axis',(0.,-1.,0.));
#35598=DIRECTION('ref_axis',(1.,0.,0.));
#35599=DIRECTION('',(0.122161987175083,0.,-0.992510175710776));
#35600=DIRECTION('center_axis',(-0.992510175710776,0.,-0.122161987175083));
#35601=DIRECTION('ref_axis',(-0.122161987175083,0.,0.992510175710776));
#35602=DIRECTION('',(0.,1.,0.));
#35603=DIRECTION('',(-0.122161987175083,0.,0.992510175710776));
#35604=DIRECTION('center_axis',(0.,1.,0.));
#35605=DIRECTION('ref_axis',(-0.951056516295154,0.,0.309016994374948));
#35606=DIRECTION('center_axis',(0.,1.,0.));
#35607=DIRECTION('ref_axis',(1.,0.,0.));
#35608=DIRECTION('center_axis',(0.615429106107016,0.,-0.788192245176467));
#35609=DIRECTION('ref_axis',(-0.788192245176467,0.,-0.615429106107016));
#35610=DIRECTION('',(0.,-1.,0.));
#35611=DIRECTION('',(-0.788192245176467,0.,-0.615429106107016));
#35612=DIRECTION('',(0.,1.,0.));
#35613=DIRECTION('',(0.788192245176467,0.,0.615429106107016));
#35614=DIRECTION('center_axis',(0.,1.,0.));
#35615=DIRECTION('ref_axis',(0.453990499739547,0.,0.891006524188368));
#35616=DIRECTION('center_axis',(0.,-1.,0.));
#35617=DIRECTION('ref_axis',(1.,0.,0.));
#35618=DIRECTION('',(-0.0346048279875384,0.,-0.99940107358355));
#35619=DIRECTION('center_axis',(-0.99940107358355,0.,0.0346048279875384));
#35620=DIRECTION('ref_axis',(0.0346048279875384,0.,0.99940107358355));
#35621=DIRECTION('',(0.,1.,0.));
#35622=DIRECTION('',(0.0346048279875384,0.,0.99940107358355));
#35623=DIRECTION('center_axis',(0.,1.,0.));
#35624=DIRECTION('ref_axis',(-0.891006524188368,0.,0.453990499739547));
#35625=DIRECTION('center_axis',(0.,1.,0.));
#35626=DIRECTION('ref_axis',(1.,0.,0.));
#35627=DIRECTION('center_axis',(0.484551720341748,0.,-0.874762613692339));
#35628=DIRECTION('ref_axis',(-0.874762613692339,0.,-0.484551720341748));
#35629=DIRECTION('',(0.,-1.,0.));
#35630=DIRECTION('',(-0.874762613692339,0.,-0.484551720341748));
#35631=DIRECTION('',(0.,1.,0.));
#35632=DIRECTION('',(0.874762613692339,0.,0.484551720341748));
#35633=DIRECTION('center_axis',(0.,1.,0.));
#35634=DIRECTION('ref_axis',(0.587785252292473,0.,0.809016994374947));
#35635=DIRECTION('center_axis',(0.,-1.,0.));
#35636=DIRECTION('ref_axis',(1.,0.,0.));
#35637=DIRECTION('',(-0.190519557438267,0.,-0.981683400202696));
#35638=DIRECTION('center_axis',(-0.981683400202696,0.,0.190519557438267));
#35639=DIRECTION('ref_axis',(0.190519557438267,0.,0.981683400202696));
#35640=DIRECTION('',(0.,1.,0.));
#35641=DIRECTION('',(0.190519557438267,0.,0.981683400202696));
#35642=DIRECTION('center_axis',(0.,1.,0.));
#35643=DIRECTION('ref_axis',(-0.809016994374947,0.,0.587785252292473));
#35644=DIRECTION('center_axis',(0.,1.,0.));
#35645=DIRECTION('ref_axis',(1.,0.,0.));
#35646=DIRECTION('center_axis',(0.341743063086706,0.,-0.939793423488437));
#35647=DIRECTION('ref_axis',(-0.939793423488437,0.,-0.341743063086706));
#35648=DIRECTION('',(0.,-1.,0.));
#35649=DIRECTION('',(-0.939793423488437,0.,-0.341743063086706));
#35650=DIRECTION('',(0.,1.,0.));
#35651=DIRECTION('',(0.939793423488437,0.,0.341743063086706));
#35652=DIRECTION('center_axis',(0.,1.,0.));
#35653=DIRECTION('ref_axis',(0.707106781186548,0.,0.707106781186548));
#35654=DIRECTION('center_axis',(0.,-1.,0.));
#35655=DIRECTION('ref_axis',(1.,0.,0.));
#35656=DIRECTION('',(-0.341743063086706,0.,-0.939793423488437));
#35657=DIRECTION('center_axis',(-0.939793423488437,0.,0.341743063086706));
#35658=DIRECTION('ref_axis',(0.341743063086706,0.,0.939793423488437));
#35659=DIRECTION('',(0.,1.,0.));
#35660=DIRECTION('',(0.341743063086706,0.,0.939793423488437));
#35661=DIRECTION('center_axis',(0.,1.,0.));
#35662=DIRECTION('ref_axis',(-0.707106781186548,0.,0.707106781186548));
#35663=DIRECTION('center_axis',(0.,1.,0.));
#35664=DIRECTION('ref_axis',(1.,0.,0.));
#35665=DIRECTION('center_axis',(0.190519557438267,0.,-0.981683400202696));
#35666=DIRECTION('ref_axis',(-0.981683400202696,0.,-0.190519557438267));
#35667=DIRECTION('',(0.,-1.,0.));
#35668=DIRECTION('',(-0.981683400202696,0.,-0.190519557438267));
#35669=DIRECTION('',(0.,1.,0.));
#35670=DIRECTION('',(0.981683400202696,0.,0.190519557438267));
#35671=DIRECTION('center_axis',(0.,1.,0.));
#35672=DIRECTION('ref_axis',(0.809016994374947,0.,0.587785252292473));
#35673=DIRECTION('center_axis',(0.,-1.,0.));
#35674=DIRECTION('ref_axis',(1.,0.,0.));
#35675=DIRECTION('',(-0.484551720341748,0.,-0.874762613692339));
#35676=DIRECTION('center_axis',(-0.874762613692339,0.,0.484551720341748));
#35677=DIRECTION('ref_axis',(0.484551720341748,0.,0.874762613692339));
#35678=DIRECTION('',(0.,1.,0.));
#35679=DIRECTION('',(0.484551720341748,0.,0.874762613692339));
#35680=DIRECTION('center_axis',(0.,1.,0.));
#35681=DIRECTION('ref_axis',(-0.587785252292473,0.,0.809016994374947));
#35682=DIRECTION('center_axis',(0.,1.,0.));
#35683=DIRECTION('ref_axis',(1.,0.,0.));
#35684=DIRECTION('center_axis',(0.0346048279875382,0.,-0.99940107358355));
#35685=DIRECTION('ref_axis',(-0.99940107358355,0.,-0.0346048279875382));
#35686=DIRECTION('',(0.,-1.,0.));
#35687=DIRECTION('',(-0.99940107358355,0.,-0.0346048279875382));
#35688=DIRECTION('',(0.,1.,0.));
#35689=DIRECTION('',(0.99940107358355,0.,0.0346048279875382));
#35690=DIRECTION('center_axis',(0.,1.,0.));
#35691=DIRECTION('ref_axis',(0.891006524188368,0.,0.453990499739547));
#35692=DIRECTION('center_axis',(0.,-1.,0.));
#35693=DIRECTION('ref_axis',(1.,0.,0.));
#35694=DIRECTION('',(-0.615429106107016,0.,-0.788192245176467));
#35695=DIRECTION('center_axis',(-0.788192245176467,0.,0.615429106107016));
#35696=DIRECTION('ref_axis',(0.615429106107016,0.,0.788192245176467));
#35697=DIRECTION('',(0.,1.,0.));
#35698=DIRECTION('',(0.615429106107016,0.,0.788192245176467));
#35699=DIRECTION('center_axis',(0.,1.,0.));
#35700=DIRECTION('ref_axis',(-0.453990499739547,0.,0.891006524188368));
#35701=DIRECTION('center_axis',(0.,1.,0.));
#35702=DIRECTION('ref_axis',(1.,0.,0.));
#35703=DIRECTION('center_axis',(-0.122161987175083,0.,-0.992510175710776));
#35704=DIRECTION('ref_axis',(-0.992510175710776,0.,0.122161987175083));
#35705=DIRECTION('',(0.,-1.,0.));
#35706=DIRECTION('',(-0.992510175710776,0.,0.122161987175083));
#35707=DIRECTION('',(0.,1.,0.));
#35708=DIRECTION('',(0.992510175710776,0.,-0.122161987175083));
#35709=DIRECTION('center_axis',(0.,1.,0.));
#35710=DIRECTION('ref_axis',(0.951056516295154,0.,0.309016994374947));
#35711=DIRECTION('center_axis',(0.,-1.,0.));
#35712=DIRECTION('ref_axis',(1.,0.,0.));
#35713=DIRECTION('',(-0.731152584787826,0.,-0.682213967724262));
#35714=DIRECTION('center_axis',(-0.682213967724262,0.,0.731152584787827));
#35715=DIRECTION('ref_axis',(0.731152584787827,0.,0.682213967724262));
#35716=DIRECTION('',(0.,1.,0.));
#35717=DIRECTION('',(0.731152584787826,0.,0.682213967724262));
#35718=DIRECTION('center_axis',(0.,1.,0.));
#35719=DIRECTION('ref_axis',(-0.309016994374947,0.,0.951056516295154));
#35720=DIRECTION('center_axis',(0.,1.,0.));
#35721=DIRECTION('ref_axis',(1.,0.,0.));
#35722=DIRECTION('center_axis',(-0.275920768781063,0.,-0.961180383359579));
#35723=DIRECTION('ref_axis',(-0.961180383359579,0.,0.275920768781063));
#35724=DIRECTION('',(0.,-1.,0.));
#35725=DIRECTION('',(-0.961180383359579,0.,0.275920768781063));
#35726=DIRECTION('',(0.,1.,0.));
#35727=DIRECTION('center_axis',(0.,1.,0.));
#35728=DIRECTION('ref_axis',(0.987688340595138,0.,0.156434465040231));
#35729=DIRECTION('center_axis',(0.,-1.,0.));
#35730=DIRECTION('ref_axis',(1.,0.,0.));
#35731=DIRECTION('center_axis',(-0.559437318248335,0.,0.828872660274852));
#35732=DIRECTION('ref_axis',(0.828872660274852,0.,0.559437318248335));
#35733=DIRECTION('',(0.828872660274852,0.,0.559437318248335));
#35734=DIRECTION('',(0.,1.,0.));
#35735=DIRECTION('center_axis',(0.,1.,0.));
#35736=DIRECTION('ref_axis',(-0.156434465040231,0.,0.987688340595138));
#35737=DIRECTION('center_axis',(0.,1.,0.));
#35738=DIRECTION('ref_axis',(1.,0.,0.));
#35739=DIRECTION('center_axis',(0.,1.,0.));
#35740=DIRECTION('ref_axis',(1.,0.,0.));
#35741=DIRECTION('center_axis',(0.,-1.,0.));
#35742=DIRECTION('ref_axis',(1.,0.,0.));
#35743=DIRECTION('center_axis',(0.,1.,0.));
#35744=DIRECTION('ref_axis',(0.,0.,1.));
#35745=DIRECTION('center_axis',(0.,1.,0.));
#35746=DIRECTION('ref_axis',(1.,0.,0.));
#35747=DIRECTION('center_axis',(0.,1.,0.));
#35748=DIRECTION('ref_axis',(1.,0.,0.));
#35749=DIRECTION('center_axis',(0.,1.,0.));
#35750=DIRECTION('ref_axis',(1.,0.,0.));
#35751=DIRECTION('',(-0.991409720169891,0.130792839072551,1.21412674044963E-16));
#35752=DIRECTION('center_axis',(0.,-1.,0.));
#35753=DIRECTION('ref_axis',(1.,0.,0.));
#35754=DIRECTION('center_axis',(0.,1.,0.));
#35755=DIRECTION('ref_axis',(0.,0.,1.));
#35756=DIRECTION('center_axis',(0.,-1.,0.));
#35757=DIRECTION('ref_axis',(1.,0.,0.));
#35758=DIRECTION('center_axis',(0.,-1.,0.));
#35759=DIRECTION('ref_axis',(1.,0.,0.));
#35760=DIRECTION('center_axis',(0.,-1.,0.));
#35761=DIRECTION('ref_axis',(1.,0.,0.));
#35762=DIRECTION('',(0.707106781186544,0.707106781186551,8.6595605623549E-17));
#35763=DIRECTION('center_axis',(0.,-1.,0.));
#35764=DIRECTION('ref_axis',(1.,0.,0.));
#35765=DIRECTION('center_axis',(0.,-1.,0.));
#35766=DIRECTION('ref_axis',(1.,0.,0.));
#35767=DIRECTION('',(0.,1.,0.));
#35768=DIRECTION('',(0.,1.,0.));
#35769=DIRECTION('center_axis',(0.,1.,0.));
#35770=DIRECTION('ref_axis',(1.,0.,0.));
#35771=DIRECTION('',(0.707106781186539,-0.707106781186556,-8.65956056235483E-17));
#35772=DIRECTION('center_axis',(0.,-1.,0.));
#35773=DIRECTION('ref_axis',(1.,0.,0.));
#35774=DIRECTION('center_axis',(0.,-1.,0.));
#35775=DIRECTION('ref_axis',(0.,0.,-1.));
#35776=DIRECTION('center_axis',(0.,-1.,0.));
#35777=DIRECTION('ref_axis',(1.,0.,0.));
#35778=DIRECTION('center_axis',(0.,-1.,0.));
#35779=DIRECTION('ref_axis',(1.,0.,0.));
#35780=DIRECTION('center_axis',(0.,-1.,0.));
#35781=DIRECTION('ref_axis',(1.,0.,0.));
#35782=DIRECTION('',(0.,1.,0.));
#35783=DIRECTION('center_axis',(0.,-1.,0.));
#35784=DIRECTION('ref_axis',(0.,0.,-1.));
#35785=DIRECTION('center_axis',(0.,-1.,0.));
#35786=DIRECTION('ref_axis',(1.,0.,0.));
#35787=DIRECTION('center_axis',(0.,-1.,0.));
#35788=DIRECTION('ref_axis',(1.,0.,0.));
#35789=DIRECTION('',(0.,-1.,0.));
#69010=CARTESIAN_POINT('',(0.,0.,0.));
#69011=CARTESIAN_POINT('Origin',(8.,139.,13.3));
#69012=CARTESIAN_POINT('',(7.37215620887551,138.292054261923,14.6788810071715));
#69013=CARTESIAN_POINT('',(7.33808558140337,139.,14.85));
#69014=CARTESIAN_POINT('Ctrl Pts',(7.37215620887549,138.292054261923,14.6788810071716));
#69015=CARTESIAN_POINT('Ctrl Pts',(7.36858316305761,138.329261989146,14.697984216059));
#69016=CARTESIAN_POINT('Ctrl Pts',(7.36520732362226,138.367331819182,14.7156231689265));
#69017=CARTESIAN_POINT('Ctrl Pts',(7.3466854762311,138.596916234109,14.8108668747228));
#69018=CARTESIAN_POINT('Ctrl Pts',(7.33808558140337,138.804765733125,14.85));
#69019=CARTESIAN_POINT('Ctrl Pts',(7.33808558140337,139.,14.85));
#69020=CARTESIAN_POINT('',(6.96320280119572,137.910875006907,14.4028629785336));
#69021=CARTESIAN_POINT('Origin',(5.32918064872639,139.,13.3));
#69022=CARTESIAN_POINT('',(7.43743486603367,137.788415340765,14.2667277866632));
#69023=CARTESIAN_POINT('Origin',(10.8050674972932,139.,13.3));
#69024=CARTESIAN_POINT('',(7.4970972452634,137.464107065927,13.5086453811229));
#69025=CARTESIAN_POINT('Ctrl Pts',(7.4970972452634,137.464107065927,13.5086453811229));
#69026=CARTESIAN_POINT('Ctrl Pts',(7.49347284068085,137.481798737663,13.6388783796458));
#69027=CARTESIAN_POINT('Ctrl Pts',(7.48629498464008,137.516874519344,13.7699539370805));
#69028=CARTESIAN_POINT('Ctrl Pts',(7.46572064431159,137.624316026987,14.0289417164261));
#69029=CARTESIAN_POINT('Ctrl Pts',(7.45185181981712,137.699915413076,14.1558122257263));
#69030=CARTESIAN_POINT('Ctrl Pts',(7.43743486603368,137.788415340765,14.2667277866631));
#69031=CARTESIAN_POINT('',(7.05,137.45,13.3));
#69032=CARTESIAN_POINT('Origin',(7.05,139.,13.3));
#69033=CARTESIAN_POINT('',(7.4970972452634,137.464107065927,13.0913546188771));
#69034=CARTESIAN_POINT('Origin',(7.05,139.,13.3));
#69035=CARTESIAN_POINT('',(7.43743486603367,137.788415340765,12.3332722133368));
#69036=CARTESIAN_POINT('Ctrl Pts',(7.43743486603368,137.788415340765,12.3332722133368));
#69037=CARTESIAN_POINT('Ctrl Pts',(7.45185181981712,137.699915413076,12.4441877742737));
#69038=CARTESIAN_POINT('Ctrl Pts',(7.46572064431159,137.624316026987,12.5710582835739));
#69039=CARTESIAN_POINT('Ctrl Pts',(7.48629498464007,137.516874519344,12.8300460629195));
#69040=CARTESIAN_POINT('Ctrl Pts',(7.49347284068085,137.481798737663,12.9611216203542));
#69041=CARTESIAN_POINT('Ctrl Pts',(7.4970972452634,137.464107065927,13.0913546188771));
#69042=CARTESIAN_POINT('',(6.96320280119572,137.910875006907,12.1971370214664));
#69043=CARTESIAN_POINT('Origin',(10.8050674972932,139.,13.3));
#69044=CARTESIAN_POINT('',(7.37215620887551,138.292054261923,11.9211189928285));
#69045=CARTESIAN_POINT('Origin',(5.32918064872639,139.,13.3));
#69046=CARTESIAN_POINT('',(7.37215620887551,139.707945738077,11.9211189928285));
#69047=CARTESIAN_POINT('Ctrl Pts',(7.37215620887549,139.707945738077,11.9211189928284));
#69048=CARTESIAN_POINT('Ctrl Pts',(7.36858316305761,139.670738010854,11.902015783941));
#69049=CARTESIAN_POINT('Ctrl Pts',(7.36520732362226,139.632668180818,11.8843768310735));
#69050=CARTESIAN_POINT('Ctrl Pts',(7.3466854762311,139.403083765891,11.7891331252772));
#69051=CARTESIAN_POINT('Ctrl Pts',(7.33808558140337,139.195234266875,11.75));
#69052=CARTESIAN_POINT('Ctrl Pts',(7.33808558140337,139.,11.75));
#69053=CARTESIAN_POINT('Ctrl Pts',(7.33808558140337,138.804765733125,11.75));
#69054=CARTESIAN_POINT('Ctrl Pts',(7.3466854762311,138.596916234109,11.7891331252772));
#69055=CARTESIAN_POINT('Ctrl Pts',(7.36520732362226,138.367331819182,11.8843768310735));
#69056=CARTESIAN_POINT('Ctrl Pts',(7.36858316305761,138.329261989146,11.902015783941));
#69057=CARTESIAN_POINT('Ctrl Pts',(7.37215620887549,138.292054261923,11.9211189928284));
#69058=CARTESIAN_POINT('',(6.96320280119572,140.089124993093,12.1971370214664));
#69059=CARTESIAN_POINT('Origin',(5.32918064872639,139.,13.3));
#69060=CARTESIAN_POINT('',(7.43743486603367,140.211584659235,12.3332722133368));
#69061=CARTESIAN_POINT('Origin',(10.8050674972932,139.,13.3));
#69062=CARTESIAN_POINT('',(7.4970972452634,140.535892934073,13.0913546188771));
#69063=CARTESIAN_POINT('Ctrl Pts',(7.4970972452634,140.535892934073,13.0913546188771));
#69064=CARTESIAN_POINT('Ctrl Pts',(7.49347284068085,140.518201262337,12.9611216203542));
#69065=CARTESIAN_POINT('Ctrl Pts',(7.48629498464008,140.483125480656,12.8300460629195));
#69066=CARTESIAN_POINT('Ctrl Pts',(7.46572064431159,140.375683973014,12.5710582835739));
#69067=CARTESIAN_POINT('Ctrl Pts',(7.45185181981713,140.300084586924,12.4441877742737));
#69068=CARTESIAN_POINT('Ctrl Pts',(7.43743486603368,140.211584659235,12.3332722133369));
#69069=CARTESIAN_POINT('',(7.05,140.55,13.3));
#69070=CARTESIAN_POINT('Origin',(7.05,139.,13.3));
#69071=CARTESIAN_POINT('',(7.4970972452634,140.535892934073,13.5086453811229));
#69072=CARTESIAN_POINT('Origin',(7.05,139.,13.3));
#69073=CARTESIAN_POINT('',(7.43743486603367,140.211584659235,14.2667277866632));
#69074=CARTESIAN_POINT('Ctrl Pts',(7.43743486603368,140.211584659235,14.2667277866631));
#69075=CARTESIAN_POINT('Ctrl Pts',(7.45185181981713,140.300084586924,14.1558122257262));
#69076=CARTESIAN_POINT('Ctrl Pts',(7.46572064431159,140.375683973013,14.0289417164261));
#69077=CARTESIAN_POINT('Ctrl Pts',(7.48629498464008,140.483125480656,13.7699539370805));
#69078=CARTESIAN_POINT('Ctrl Pts',(7.49347284068085,140.518201262337,13.6388783796458));
#69079=CARTESIAN_POINT('Ctrl Pts',(7.4970972452634,140.535892934073,13.5086453811229));
#69080=CARTESIAN_POINT('',(6.96320280119572,140.089124993093,14.4028629785336));
#69081=CARTESIAN_POINT('Origin',(10.8050674972932,139.,13.3));
#69082=CARTESIAN_POINT('',(7.37215620887551,139.707945738077,14.6788810071715));
#69083=CARTESIAN_POINT('Origin',(5.32918064872639,139.,13.3));
#69084=CARTESIAN_POINT('Ctrl Pts',(7.33808558140337,139.,14.85));
#69085=CARTESIAN_POINT('Ctrl Pts',(7.33808558140337,139.195234266875,14.85));
#69086=CARTESIAN_POINT('Ctrl Pts',(7.3466854762311,139.403083765891,14.8108668747228));
#69087=CARTESIAN_POINT('Ctrl Pts',(7.36520732362226,139.632668180818,14.7156231689265));
#69088=CARTESIAN_POINT('Ctrl Pts',(7.36858316305761,139.670738010854,14.697984216059));
#69089=CARTESIAN_POINT('Ctrl Pts',(7.37215620887549,139.707945738077,14.6788810071716));
#69090=CARTESIAN_POINT('',(1.27968746184371,139.,14.85));
#69091=CARTESIAN_POINT('',(8.,139.,14.85));
#69092=CARTESIAN_POINT('',(1.27968746184371,139.,11.75));
#69093=CARTESIAN_POINT('Ctrl Pts',(1.27968746184371,139.,11.75));
#69094=CARTESIAN_POINT('Ctrl Pts',(1.27968746184371,139.104803598436,11.75));
#69095=CARTESIAN_POINT('Ctrl Pts',(1.29297627000471,139.209518837456,11.7607265104896));
#69096=CARTESIAN_POINT('Ctrl Pts',(1.34103210887612,139.413055498266,11.8024328148038));
#69097=CARTESIAN_POINT('Ctrl Pts',(1.37566593328622,139.511905723271,11.8334254159452));
#69098=CARTESIAN_POINT('Ctrl Pts',(1.49608242611994,139.793364432057,11.9529188207752));
#69099=CARTESIAN_POINT('Ctrl Pts',(1.59729725054086,139.961362416936,12.0693313952581));
#69100=CARTESIAN_POINT('Ctrl Pts',(1.7703084453967,140.227330013039,12.3352989913604));
#69101=CARTESIAN_POINT('Ctrl Pts',(1.85621230875305,140.345671919208,12.5035840227375));
#69102=CARTESIAN_POINT('Ctrl Pts',(1.97644875243109,140.507202212245,12.8835230759381));
#69103=CARTESIAN_POINT('Ctrl Pts',(2.01,140.55,13.0955898084708));
#69104=CARTESIAN_POINT('Ctrl Pts',(2.01,140.55,13.5044101915292));
#69105=CARTESIAN_POINT('Ctrl Pts',(1.97644875243109,140.507202212245,13.7164769240619));
#69106=CARTESIAN_POINT('Ctrl Pts',(1.85621230875305,140.345671919208,14.0964159772625));
#69107=CARTESIAN_POINT('Ctrl Pts',(1.7703084453967,140.227330013039,14.2647010086396));
#69108=CARTESIAN_POINT('Ctrl Pts',(1.59729725054085,139.961362416936,14.5306686047419));
#69109=CARTESIAN_POINT('Ctrl Pts',(1.49608242611994,139.793364432057,14.6470811792249));
#69110=CARTESIAN_POINT('Ctrl Pts',(1.37566593328622,139.511905723271,14.7665745840548));
#69111=CARTESIAN_POINT('Ctrl Pts',(1.34103210887612,139.413055498266,14.7975671851962));
#69112=CARTESIAN_POINT('Ctrl Pts',(1.29297627000471,139.209518837456,14.8392734895104));
#69113=CARTESIAN_POINT('Ctrl Pts',(1.27968746184371,139.104803598436,14.85));
#69114=CARTESIAN_POINT('Ctrl Pts',(1.27968746184371,139.,14.85));
#69115=CARTESIAN_POINT('Ctrl Pts',(1.27968746184371,139.,14.85));
#69116=CARTESIAN_POINT('Ctrl Pts',(1.27968746184371,138.895196401564,14.85));
#69117=CARTESIAN_POINT('Ctrl Pts',(1.29297627000471,138.790481162544,14.8392734895104));
#69118=CARTESIAN_POINT('Ctrl Pts',(1.34103210887612,138.586944501734,14.7975671851962));
#69119=CARTESIAN_POINT('Ctrl Pts',(1.37566593328622,138.488094276729,14.7665745840548));
#69120=CARTESIAN_POINT('Ctrl Pts',(1.49608242611994,138.206635567943,14.6470811792249));
#69121=CARTESIAN_POINT('Ctrl Pts',(1.59729725054086,138.038637583064,14.5306686047419));
#69122=CARTESIAN_POINT('Ctrl Pts',(1.7703084453967,137.772669986961,14.2647010086396));
#69123=CARTESIAN_POINT('Ctrl Pts',(1.85621230875305,137.654328080792,14.0964159772625));
#69124=CARTESIAN_POINT('Ctrl Pts',(1.97644875243109,137.492797787755,13.7164769240619));
#69125=CARTESIAN_POINT('Ctrl Pts',(2.01,137.45,13.5044101915292));
#69126=CARTESIAN_POINT('Ctrl Pts',(2.01,137.45,13.0955898084708));
#69127=CARTESIAN_POINT('Ctrl Pts',(1.97644875243109,137.492797787755,12.8835230759381));
#69128=CARTESIAN_POINT('Ctrl Pts',(1.85621230875305,137.654328080792,12.5035840227375));
#69129=CARTESIAN_POINT('Ctrl Pts',(1.7703084453967,137.772669986961,12.3352989913604));
#69130=CARTESIAN_POINT('Ctrl Pts',(1.59729725054086,138.038637583064,12.0693313952581));
#69131=CARTESIAN_POINT('Ctrl Pts',(1.49608242611994,138.206635567943,11.9529188207752));
#69132=CARTESIAN_POINT('Ctrl Pts',(1.37566593328622,138.488094276729,11.8334254159452));
#69133=CARTESIAN_POINT('Ctrl Pts',(1.34103210887612,138.586944501734,11.8024328148038));
#69134=CARTESIAN_POINT('Ctrl Pts',(1.29297627000471,138.790481162544,11.7607265104896));
#69135=CARTESIAN_POINT('Ctrl Pts',(1.27968746184371,138.895196401564,11.75));
#69136=CARTESIAN_POINT('Ctrl Pts',(1.27968746184371,139.,11.75));
#69137=CARTESIAN_POINT('Origin',(6.96320280119572,133.2,14.4028629785336));
#69138=CARTESIAN_POINT('',(7.37215620887551,133.2,14.6788810071715));
#69139=CARTESIAN_POINT('',(7.37215620887551,138.6,14.6788810071715));
#69140=CARTESIAN_POINT('',(6.96320280119572,133.2,14.4028629785336));
#69141=CARTESIAN_POINT('',(7.64921699387799,133.2,14.8658797465221));
#69142=CARTESIAN_POINT('',(6.96320280119572,133.2,14.4028629785336));
#69143=CARTESIAN_POINT('Origin',(7.75872111940616,133.2,14.1744979081055));
#69144=CARTESIAN_POINT('',(7.43743486603367,133.2,14.2667277866632));
#69145=CARTESIAN_POINT('',(6.96320280119572,133.2,14.4028629785336));
#69146=CARTESIAN_POINT('',(7.43743486603367,138.6,14.2667277866632));
#69147=CARTESIAN_POINT('Origin',(7.64921699387799,133.2,11.7341202534779));
#69148=CARTESIAN_POINT('',(6.96320280119572,133.2,12.1971370214664));
#69149=CARTESIAN_POINT('',(6.96320280119572,133.2,12.1971370214664));
#69150=CARTESIAN_POINT('',(7.37215620887551,133.2,11.9211189928285));
#69151=CARTESIAN_POINT('',(6.96320280119572,133.2,12.1971370214664));
#69152=CARTESIAN_POINT('',(7.37215620887551,138.6,11.9211189928285));
#69153=CARTESIAN_POINT('Origin',(7.64921699387799,133.2,11.7341202534779));
#69154=CARTESIAN_POINT('',(7.37215620887551,144.,11.9211189928285));
#69155=CARTESIAN_POINT('',(7.37215620887551,138.6,11.9211189928285));
#69156=CARTESIAN_POINT('',(6.96320280119572,144.,12.1971370214664));
#69157=CARTESIAN_POINT('',(6.96320280119572,144.,12.1971370214664));
#69158=CARTESIAN_POINT('',(6.96320280119572,133.2,12.1971370214664));
#69159=CARTESIAN_POINT('Origin',(6.96320280119572,133.2,12.1971370214664));
#69160=CARTESIAN_POINT('',(7.43743486603367,133.2,12.3332722133368));
#69161=CARTESIAN_POINT('',(7.43743486603367,138.6,12.3332722133368));
#69162=CARTESIAN_POINT('',(7.75872111940616,133.2,12.4255020918945));
#69163=CARTESIAN_POINT('Origin',(6.96320280119572,133.2,12.1971370214664));
#69164=CARTESIAN_POINT('',(7.43743486603367,144.,12.3332722133368));
#69165=CARTESIAN_POINT('',(7.75872111940616,144.,12.4255020918945));
#69166=CARTESIAN_POINT('',(7.43743486603367,138.6,12.3332722133368));
#69167=CARTESIAN_POINT('Origin',(7.05,133.2,13.3));
#69168=CARTESIAN_POINT('',(7.4970972452634,133.2,13.5086453811229));
#69169=CARTESIAN_POINT('',(7.4970972452634,138.6,13.5086453811229));
#69170=CARTESIAN_POINT('',(7.05,133.2,13.3));
#69171=CARTESIAN_POINT('',(7.8,133.2,13.65));
#69172=CARTESIAN_POINT('',(7.05,133.2,13.3));
#69173=CARTESIAN_POINT('Origin',(7.05,133.2,13.3));
#69174=CARTESIAN_POINT('',(7.05,144.,13.3));
#69175=CARTESIAN_POINT('',(7.05,133.2,13.3));
#69176=CARTESIAN_POINT('',(7.4970972452634,144.,13.5086453811229));
#69177=CARTESIAN_POINT('',(7.8,144.,13.65));
#69178=CARTESIAN_POINT('',(7.4970972452634,138.6,13.5086453811229));
#69179=CARTESIAN_POINT('Origin',(7.8,133.2,12.95));
#69180=CARTESIAN_POINT('',(7.4970972452634,133.2,13.0913546188771));
#69181=CARTESIAN_POINT('',(7.05,133.2,13.3));
#69182=CARTESIAN_POINT('',(7.4970972452634,138.6,13.0913546188771));
#69183=CARTESIAN_POINT('Origin',(7.8,133.2,12.95));
#69184=CARTESIAN_POINT('',(7.4970972452634,144.,13.0913546188771));
#69185=CARTESIAN_POINT('',(7.4970972452634,138.6,13.0913546188771));
#69186=CARTESIAN_POINT('',(7.05,144.,13.3));
#69187=CARTESIAN_POINT('Origin',(7.3335859289189,133.2,12.1384740970763));
#69188=CARTESIAN_POINT('Origin',(0.,133.2,13.3));
#69189=CARTESIAN_POINT('Origin',(7.3335859289189,144.,12.1384740970763));
#69190=CARTESIAN_POINT('Origin',(0.,144.,13.3));
#69191=CARTESIAN_POINT('Origin',(7.31008487907097,133.2,10.5567976631721));
#69192=CARTESIAN_POINT('',(7.06568821984138,144.,10.7848359934202));
#69193=CARTESIAN_POINT('',(7.06568821984138,133.2,10.7848359934202));
#69194=CARTESIAN_POINT('',(7.06568821984138,138.6,10.7848359934202));
#69195=CARTESIAN_POINT('',(6.70494843988083,144.,11.1214301896566));
#69196=CARTESIAN_POINT('',(6.70494843988083,144.,11.1214301896566));
#69197=CARTESIAN_POINT('',(6.70494843988083,133.2,11.1214301896566));
#69198=CARTESIAN_POINT('',(6.70494843988083,133.2,11.1214301896566));
#69199=CARTESIAN_POINT('',(6.70494843988083,133.2,11.1214301896566));
#69200=CARTESIAN_POINT('Origin',(7.06159463349152,133.2,11.005548816766));
#69201=CARTESIAN_POINT('',(7.19463815697102,133.2,11.1817030920438));
#69202=CARTESIAN_POINT('Origin',(0.,133.2,13.3));
#69203=CARTESIAN_POINT('',(7.52639677513343,133.2,11.2225372245787));
#69204=CARTESIAN_POINT('Origin',(6.70494843988083,133.2,11.1214301896566));
#69205=CARTESIAN_POINT('',(7.19463815697102,144.,11.1817030920438));
#69206=CARTESIAN_POINT('',(7.19463815697102,138.6,11.1817030920438));
#69207=CARTESIAN_POINT('',(7.52639677513343,144.,11.2225372245787));
#69208=CARTESIAN_POINT('Origin',(7.06159463349152,144.,11.005548816766));
#69209=CARTESIAN_POINT('Origin',(0.,144.,13.3));
#69210=CARTESIAN_POINT('Origin',(6.79095421376043,133.2,9.44702181856561));
#69211=CARTESIAN_POINT('',(6.58523953715999,144.,9.7104846792046));
#69212=CARTESIAN_POINT('',(6.58523953715999,133.2,9.7104846792046));
#69213=CARTESIAN_POINT('',(6.58523953715999,138.6,9.7104846792046));
#69214=CARTESIAN_POINT('',(6.28159599552799,144.,10.0993669768362));
#69215=CARTESIAN_POINT('',(6.28159599552799,144.,10.0993669768362));
#69216=CARTESIAN_POINT('',(6.28159599552799,133.2,10.0993669768362));
#69217=CARTESIAN_POINT('',(6.28159599552799,133.2,10.0993669768362));
#69218=CARTESIAN_POINT('',(6.28159599552799,133.2,10.0993669768362));
#69219=CARTESIAN_POINT('Origin',(6.61572344209863,133.2,9.92912053943386));
#69220=CARTESIAN_POINT('',(6.77468557884867,133.2,10.0822934708492));
#69221=CARTESIAN_POINT('Origin',(0.,133.2,13.3));
#69222=CARTESIAN_POINT('',(7.10874756357811,133.2,10.0707263854975));
#69223=CARTESIAN_POINT('Origin',(6.28159599552799,133.2,10.0993669768362));
#69224=CARTESIAN_POINT('',(6.77468557884867,144.,10.0822934708492));
#69225=CARTESIAN_POINT('',(6.77468557884867,138.6,10.0822934708492));
#69226=CARTESIAN_POINT('',(7.10874756357811,144.,10.0707263854975));
#69227=CARTESIAN_POINT('Origin',(6.61572344209863,144.,9.92912053943386));
#69228=CARTESIAN_POINT('Origin',(0.,144.,13.3));
#69229=CARTESIAN_POINT('Origin',(6.10460771782222,133.2,8.43211908408747));
#69230=CARTESIAN_POINT('',(5.9426404019167,144.,8.72451914510537));
#69231=CARTESIAN_POINT('',(5.9426404019167,133.2,8.72451914510537));
#69232=CARTESIAN_POINT('',(5.9426404019167,138.6,8.72451914510537));
#69233=CARTESIAN_POINT('',(5.70356981034338,144.,9.15611397133807));
#69234=CARTESIAN_POINT('',(5.70356981034338,144.,9.15611397133807));
#69235=CARTESIAN_POINT('',(5.70356981034338,133.2,9.15611397133807));
#69236=CARTESIAN_POINT('',(5.70356981034338,133.2,9.15611397133807));
#69237=CARTESIAN_POINT('',(5.70356981034338,133.2,9.15611397133807));
#69238=CARTESIAN_POINT('Origin',(6.00695118323399,133.2,8.93569450172839));
#69239=CARTESIAN_POINT('',(6.18791775788269,133.2,9.06211446335793));
#69240=CARTESIAN_POINT('Origin',(0.,133.2,13.3));
#69241=CARTESIAN_POINT('',(6.51605739442695,133.2,8.99843098014994));
#69242=CARTESIAN_POINT('Origin',(5.70356981034338,133.2,9.15611397133807));
#69243=CARTESIAN_POINT('',(6.18791775788269,144.,9.06211446335793));
#69244=CARTESIAN_POINT('',(6.18791775788269,138.6,9.06211446335793));
#69245=CARTESIAN_POINT('',(6.51605739442695,144.,8.99843098014994));
#69246=CARTESIAN_POINT('Origin',(6.00695118323399,144.,8.93569450172839));
#69247=CARTESIAN_POINT('Origin',(0.,144.,13.3));
#69248=CARTESIAN_POINT('Origin',(5.26794551983978,133.2,7.53707973332964));
#69249=CARTESIAN_POINT('',(5.15371373748547,144.,7.851217134804));
#69250=CARTESIAN_POINT('',(5.15371373748547,133.2,7.851217134804));
#69251=CARTESIAN_POINT('',(5.15371373748547,138.6,7.851217134804));
#69252=CARTESIAN_POINT('',(4.98510280736516,144.,8.31489719263484));
#69253=CARTESIAN_POINT('',(4.98510280736516,144.,8.31489719263484));
#69254=CARTESIAN_POINT('',(4.98510280736516,133.2,8.31489719263484));
#69255=CARTESIAN_POINT('',(4.98510280736516,133.2,8.31489719263484));
#69256=CARTESIAN_POINT('',(4.98510280736516,133.2,8.31489719263484));
#69257=CARTESIAN_POINT('Origin',(5.25026785031011,133.2,8.04973214968988));
#69258=CARTESIAN_POINT('',(5.448782865196,133.2,8.14628626251453));
#69259=CARTESIAN_POINT('Origin',(0.,133.2,13.3));
#69260=CARTESIAN_POINT('',(5.76292026667036,133.2,8.03205448016022));
#69261=CARTESIAN_POINT('Origin',(4.98510280736516,133.2,8.31489719263484));
#69262=CARTESIAN_POINT('',(5.448782865196,144.,8.14628626251453));
#69263=CARTESIAN_POINT('',(5.448782865196,138.6,8.14628626251453));
#69264=CARTESIAN_POINT('',(5.76292026667036,144.,8.03205448016022));
#69265=CARTESIAN_POINT('Origin',(5.25026785031011,144.,8.04973214968988));
#69266=CARTESIAN_POINT('Origin',(0.,144.,13.3));
#69267=CARTESIAN_POINT('Origin',(4.30156901985006,133.2,6.78394260557304));
#69268=CARTESIAN_POINT('',(4.23788553664207,144.,7.11208224211731));
#69269=CARTESIAN_POINT('',(4.23788553664207,133.2,7.11208224211731));
#69270=CARTESIAN_POINT('',(4.23788553664207,138.6,7.11208224211731));
#69271=CARTESIAN_POINT('',(4.14388602866193,144.,7.59643018965662));
#69272=CARTESIAN_POINT('',(4.14388602866193,144.,7.59643018965662));
#69273=CARTESIAN_POINT('',(4.14388602866193,133.2,7.59643018965662));
#69274=CARTESIAN_POINT('',(4.14388602866193,133.2,7.59643018965662));
#69275=CARTESIAN_POINT('',(4.14388602866193,133.2,7.59643018965662));
#69276=CARTESIAN_POINT('Origin',(4.36430549827161,133.2,7.29304881676602));
#69277=CARTESIAN_POINT('',(4.57548085489463,133.2,7.3573595980833));
#69278=CARTESIAN_POINT('Origin',(0.,133.2,13.3));
#69279=CARTESIAN_POINT('',(4.86788091591252,133.2,7.19539228217777));
#69280=CARTESIAN_POINT('Origin',(4.14388602866193,133.2,7.59643018965662));
#69281=CARTESIAN_POINT('',(4.57548085489463,144.,7.3573595980833));
#69282=CARTESIAN_POINT('',(4.57548085489463,138.6,7.3573595980833));
#69283=CARTESIAN_POINT('',(4.86788091591252,144.,7.19539228217777));
#69284=CARTESIAN_POINT('Origin',(4.36430549827161,144.,7.29304881676602));
#69285=CARTESIAN_POINT('Origin',(0.,144.,13.3));
#69286=CARTESIAN_POINT('Origin',(3.22927361450254,133.2,6.19125243642189));
#69287=CARTESIAN_POINT('',(3.21770652915082,144.,6.52531442115133));
#69288=CARTESIAN_POINT('',(3.21770652915082,133.2,6.52531442115133));
#69289=CARTESIAN_POINT('',(3.21770652915082,138.6,6.52531442115133));
#69290=CARTESIAN_POINT('',(3.2006330231638,144.,7.01840400447201));
#69291=CARTESIAN_POINT('',(3.2006330231638,144.,7.01840400447201));
#69292=CARTESIAN_POINT('',(3.2006330231638,133.2,7.01840400447201));
#69293=CARTESIAN_POINT('',(3.2006330231638,133.2,7.01840400447201));
#69294=CARTESIAN_POINT('',(3.2006330231638,133.2,7.01840400447201));
#69295=CARTESIAN_POINT('Origin',(3.37087946056613,133.2,6.68427655790137));
#69296=CARTESIAN_POINT('',(3.5895153207954,133.2,6.71476046284001));
#69297=CARTESIAN_POINT('Origin',(0.,133.2,13.3));
#69298=CARTESIAN_POINT('',(3.85297818143439,133.2,6.50904578623957));
#69299=CARTESIAN_POINT('Origin',(3.2006330231638,133.2,7.01840400447201));
#69300=CARTESIAN_POINT('',(3.5895153207954,144.,6.71476046284001));
#69301=CARTESIAN_POINT('',(3.5895153207954,138.6,6.71476046284001));
#69302=CARTESIAN_POINT('',(3.85297818143439,144.,6.50904578623957));
#69303=CARTESIAN_POINT('Origin',(3.37087946056613,144.,6.68427655790137));
#69304=CARTESIAN_POINT('Origin',(0.,144.,13.3));
#69305=CARTESIAN_POINT('Origin',(2.07746277542129,133.2,5.77360322486657));
#69306=CARTESIAN_POINT('',(2.11829690795615,144.,6.10536184302898));
#69307=CARTESIAN_POINT('',(2.11829690795615,133.2,6.10536184302898));
#69308=CARTESIAN_POINT('',(2.11829690795615,138.6,6.10536184302898));
#69309=CARTESIAN_POINT('',(2.17856981034338,144.,6.59505156011917));
#69310=CARTESIAN_POINT('',(2.17856981034338,144.,6.59505156011917));
#69311=CARTESIAN_POINT('',(2.17856981034338,133.2,6.59505156011917));
#69312=CARTESIAN_POINT('',(2.17856981034338,133.2,6.59505156011917));
#69313=CARTESIAN_POINT('',(2.17856981034338,133.2,6.59505156011917));
#69314=CARTESIAN_POINT('Origin',(2.29445118323398,133.2,6.23840536650849));
#69315=CARTESIAN_POINT('',(2.51516400657983,133.2,6.23431178015862));
#69316=CARTESIAN_POINT('Origin',(0.,133.2,13.3));
#69317=CARTESIAN_POINT('',(2.74320233682789,133.2,5.98991512092903));
#69318=CARTESIAN_POINT('Origin',(2.17856981034338,133.2,6.59505156011917));
#69319=CARTESIAN_POINT('',(2.51516400657983,144.,6.23431178015862));
#69320=CARTESIAN_POINT('',(2.51516400657983,138.6,6.23431178015862));
#69321=CARTESIAN_POINT('',(2.74320233682789,144.,5.98991512092903));
#69322=CARTESIAN_POINT('Origin',(2.29445118323398,144.,6.23840536650849));
#69323=CARTESIAN_POINT('Origin',(0.,144.,13.3));
#69324=CARTESIAN_POINT('Origin',(0.874497908105503,133.2,5.54127888059385));
#69325=CARTESIAN_POINT('',(0.96672778666323,144.,5.86256513396634));
#69326=CARTESIAN_POINT('',(0.96672778666323,133.2,5.86256513396634));
#69327=CARTESIAN_POINT('',(0.966727786663231,138.6,5.86256513396633));
#69328=CARTESIAN_POINT('',(1.10286297853363,144.,6.33679719880428));
#69329=CARTESIAN_POINT('',(1.10286297853363,144.,6.33679719880428));
#69330=CARTESIAN_POINT('',(1.10286297853363,133.2,6.33679719880428));
#69331=CARTESIAN_POINT('',(1.10286297853363,133.2,6.33679719880428));
#69332=CARTESIAN_POINT('',(1.10286297853363,133.2,6.33679719880428));
#69333=CARTESIAN_POINT('Origin',(1.16152590292371,133.2,5.9664140710811));
#69334=CARTESIAN_POINT('',(1.37888100717151,133.2,5.92784379112449));
#69335=CARTESIAN_POINT('Origin',(0.,133.2,13.3));
#69336=CARTESIAN_POINT('',(1.5658797465221,133.2,5.65078300612201));
#69337=CARTESIAN_POINT('Origin',(1.10286297853363,133.2,6.33679719880428));
#69338=CARTESIAN_POINT('',(1.37888100717151,144.,5.92784379112449));
#69339=CARTESIAN_POINT('',(1.3788810071715,138.6,5.92784379112449));
#69340=CARTESIAN_POINT('',(1.5658797465221,144.,5.65078300612201));
#69341=CARTESIAN_POINT('Origin',(1.16152590292371,144.,5.9664140710811));
#69342=CARTESIAN_POINT('Origin',(0.,144.,13.3));
#69343=CARTESIAN_POINT('Origin',(-0.350000000000001,133.2,5.5));
#69344=CARTESIAN_POINT('',(-0.208645381122922,144.,5.8029027547366));
#69345=CARTESIAN_POINT('',(-0.208645381122922,133.2,5.8029027547366));
#69346=CARTESIAN_POINT('',(-0.208645381122922,138.6,5.8029027547366));
#69347=CARTESIAN_POINT('',(-2.22044604925031E-15,144.,6.25));
#69348=CARTESIAN_POINT('',(-2.22044604925031E-15,144.,6.25));
#69349=CARTESIAN_POINT('',(-2.22044604925031E-15,133.2,6.25));
#69350=CARTESIAN_POINT('',(-2.22044604925031E-15,133.2,6.25));
#69351=CARTESIAN_POINT('',(-2.22044604925031E-15,133.2,6.25));
#69352=CARTESIAN_POINT('Origin',(-2.22044604925031E-15,133.2,5.875));
#69353=CARTESIAN_POINT('',(0.208645381122917,133.2,5.8029027547366));
#69354=CARTESIAN_POINT('Origin',(0.,133.2,13.3));
#69355=CARTESIAN_POINT('',(0.349999999999997,133.2,5.5));
#69356=CARTESIAN_POINT('Origin',(-2.22044604925031E-15,133.2,6.25));
#69357=CARTESIAN_POINT('',(0.208645381122917,144.,5.8029027547366));
#69358=CARTESIAN_POINT('',(0.208645381122917,138.6,5.8029027547366));
#69359=CARTESIAN_POINT('',(0.349999999999997,144.,5.5));
#69360=CARTESIAN_POINT('Origin',(-2.22044604925031E-15,144.,5.875));
#69361=CARTESIAN_POINT('Origin',(0.,144.,13.3));
#69362=CARTESIAN_POINT('Origin',(-1.5658797465221,133.2,5.65078300612201));
#69363=CARTESIAN_POINT('',(-1.37888100717151,144.,5.92784379112449));
#69364=CARTESIAN_POINT('',(-1.37888100717151,133.2,5.92784379112449));
#69365=CARTESIAN_POINT('',(-1.37888100717151,138.6,5.92784379112449));
#69366=CARTESIAN_POINT('',(-1.10286297853363,144.,6.33679719880428));
#69367=CARTESIAN_POINT('',(-1.10286297853363,144.,6.33679719880428));
#69368=CARTESIAN_POINT('',(-1.10286297853363,133.2,6.33679719880428));
#69369=CARTESIAN_POINT('',(-1.10286297853363,133.2,6.33679719880428));
#69370=CARTESIAN_POINT('',(-1.10286297853363,133.2,6.33679719880428));
#69371=CARTESIAN_POINT('Origin',(-1.16152590292371,133.2,5.9664140710811));
#69372=CARTESIAN_POINT('',(-0.966727786663231,133.2,5.86256513396633));
#69373=CARTESIAN_POINT('Origin',(0.,133.2,13.3));
#69374=CARTESIAN_POINT('',(-0.874497908105503,133.2,5.54127888059384));
#69375=CARTESIAN_POINT('Origin',(-1.10286297853363,133.2,6.33679719880428));
#69376=CARTESIAN_POINT('',(-0.966727786663231,144.,5.86256513396633));
#69377=CARTESIAN_POINT('',(-0.966727786663235,138.6,5.86256513396633));
#69378=CARTESIAN_POINT('',(-0.874497908105503,144.,5.54127888059384));
#69379=CARTESIAN_POINT('Origin',(-1.16152590292371,144.,5.9664140710811));
#69380=CARTESIAN_POINT('Origin',(0.,144.,13.3));
#69381=CARTESIAN_POINT('Origin',(-2.7432023368279,133.2,5.98991512092903));
#69382=CARTESIAN_POINT('',(-2.51516400657983,144.,6.23431178015862));
#69383=CARTESIAN_POINT('',(-2.51516400657983,133.2,6.23431178015862));
#69384=CARTESIAN_POINT('',(-2.51516400657984,138.6,6.23431178015862));
#69385=CARTESIAN_POINT('',(-2.17856981034338,144.,6.59505156011917));
#69386=CARTESIAN_POINT('',(-2.17856981034338,144.,6.59505156011917));
#69387=CARTESIAN_POINT('',(-2.17856981034338,133.2,6.59505156011917));
#69388=CARTESIAN_POINT('',(-2.17856981034338,133.2,6.59505156011917));
#69389=CARTESIAN_POINT('',(-2.17856981034338,133.2,6.59505156011917));
#69390=CARTESIAN_POINT('Origin',(-2.29445118323399,133.2,6.23840536650849));
#69391=CARTESIAN_POINT('',(-2.11829690795616,133.2,6.10536184302898));
#69392=CARTESIAN_POINT('Origin',(0.,133.2,13.3));
#69393=CARTESIAN_POINT('',(-2.07746277542129,133.2,5.77360322486657));
#69394=CARTESIAN_POINT('Origin',(-2.17856981034338,133.2,6.59505156011917));
#69395=CARTESIAN_POINT('',(-2.11829690795616,144.,6.10536184302898));
#69396=CARTESIAN_POINT('',(-2.11829690795616,138.6,6.10536184302898));
#69397=CARTESIAN_POINT('',(-2.07746277542129,144.,5.77360322486657));
#69398=CARTESIAN_POINT('Origin',(-2.29445118323399,144.,6.23840536650849));
#69399=CARTESIAN_POINT('Origin',(0.,144.,13.3));
#69400=CARTESIAN_POINT('Origin',(-3.85297818143439,133.2,6.50904578623957));
#69401=CARTESIAN_POINT('',(-3.5895153207954,144.,6.71476046284001));
#69402=CARTESIAN_POINT('',(-3.5895153207954,133.2,6.71476046284001));
#69403=CARTESIAN_POINT('',(-3.5895153207954,138.6,6.71476046284001));
#69404=CARTESIAN_POINT('',(-3.20063302316381,144.,7.01840400447201));
#69405=CARTESIAN_POINT('',(-3.20063302316381,144.,7.01840400447201));
#69406=CARTESIAN_POINT('',(-3.20063302316381,133.2,7.01840400447201));
#69407=CARTESIAN_POINT('',(-3.20063302316381,133.2,7.01840400447201));
#69408=CARTESIAN_POINT('',(-3.20063302316381,133.2,7.01840400447201));
#69409=CARTESIAN_POINT('Origin',(-3.37087946056614,133.2,6.68427655790137));
#69410=CARTESIAN_POINT('',(-3.21770652915082,133.2,6.52531442115133));
#69411=CARTESIAN_POINT('Origin',(0.,133.2,13.3));
#69412=CARTESIAN_POINT('',(-3.22927361450254,133.2,6.19125243642189));
#69413=CARTESIAN_POINT('Origin',(-3.20063302316381,133.2,7.01840400447201));
#69414=CARTESIAN_POINT('',(-3.21770652915082,144.,6.52531442115133));
#69415=CARTESIAN_POINT('',(-3.21770652915082,138.6,6.52531442115133));
#69416=CARTESIAN_POINT('',(-3.22927361450254,144.,6.19125243642189));
#69417=CARTESIAN_POINT('Origin',(-3.37087946056614,144.,6.68427655790137));
#69418=CARTESIAN_POINT('Origin',(0.,144.,13.3));
#69419=CARTESIAN_POINT('Origin',(-4.86788091591252,133.2,7.19539228217778));
#69420=CARTESIAN_POINT('',(-4.57548085489463,144.,7.3573595980833));
#69421=CARTESIAN_POINT('',(-4.57548085489463,133.2,7.3573595980833));
#69422=CARTESIAN_POINT('',(-4.57548085489463,138.6,7.3573595980833));
#69423=CARTESIAN_POINT('',(-4.14388602866194,144.,7.59643018965662));
#69424=CARTESIAN_POINT('',(-4.14388602866194,144.,7.59643018965662));
#69425=CARTESIAN_POINT('',(-4.14388602866194,133.2,7.59643018965662));
#69426=CARTESIAN_POINT('',(-4.14388602866194,133.2,7.59643018965662));
#69427=CARTESIAN_POINT('',(-4.14388602866194,133.2,7.59643018965662));
#69428=CARTESIAN_POINT('Origin',(-4.36430549827161,133.2,7.29304881676602));
#69429=CARTESIAN_POINT('',(-4.23788553664207,133.2,7.11208224211731));
#69430=CARTESIAN_POINT('Origin',(0.,133.2,13.3));
#69431=CARTESIAN_POINT('',(-4.30156901985006,133.2,6.78394260557305));
#69432=CARTESIAN_POINT('Origin',(-4.14388602866194,133.2,7.59643018965662));
#69433=CARTESIAN_POINT('',(-4.23788553664207,144.,7.11208224211731));
#69434=CARTESIAN_POINT('',(-4.23788553664207,138.6,7.11208224211731));
#69435=CARTESIAN_POINT('',(-4.30156901985006,144.,6.78394260557305));
#69436=CARTESIAN_POINT('Origin',(-4.36430549827161,144.,7.29304881676602));
#69437=CARTESIAN_POINT('Origin',(0.,144.,13.3));
#69438=CARTESIAN_POINT('Origin',(-5.76292026667036,133.2,8.03205448016022));
#69439=CARTESIAN_POINT('',(-5.44878286519601,144.,8.14628626251454));
#69440=CARTESIAN_POINT('',(-5.44878286519601,133.2,8.14628626251454));
#69441=CARTESIAN_POINT('',(-5.44878286519601,138.6,8.14628626251453));
#69442=CARTESIAN_POINT('',(-4.98510280736516,144.,8.31489719263484));
#69443=CARTESIAN_POINT('',(-4.98510280736516,144.,8.31489719263484));
#69444=CARTESIAN_POINT('',(-4.98510280736516,133.2,8.31489719263484));
#69445=CARTESIAN_POINT('',(-4.98510280736516,133.2,8.31489719263484));
#69446=CARTESIAN_POINT('',(-4.98510280736516,133.2,8.31489719263484));
#69447=CARTESIAN_POINT('Origin',(-5.25026785031012,133.2,8.04973214968989));
#69448=CARTESIAN_POINT('',(-5.15371373748547,133.2,7.851217134804));
#69449=CARTESIAN_POINT('Origin',(0.,133.2,13.3));
#69450=CARTESIAN_POINT('',(-5.26794551983978,133.2,7.53707973332964));
#69451=CARTESIAN_POINT('Origin',(-4.98510280736516,133.2,8.31489719263484));
#69452=CARTESIAN_POINT('',(-5.15371373748547,144.,7.851217134804));
#69453=CARTESIAN_POINT('',(-5.15371373748547,138.6,7.851217134804));
#69454=CARTESIAN_POINT('',(-5.26794551983978,144.,7.53707973332964));
#69455=CARTESIAN_POINT('Origin',(-5.25026785031012,144.,8.04973214968989));
#69456=CARTESIAN_POINT('Origin',(0.,144.,13.3));
#69457=CARTESIAN_POINT('Origin',(-6.51605739442696,133.2,8.99843098014994));
#69458=CARTESIAN_POINT('',(-6.18791775788269,144.,9.06211446335793));
#69459=CARTESIAN_POINT('',(-6.18791775788269,133.2,9.06211446335793));
#69460=CARTESIAN_POINT('',(-6.18791775788269,138.6,9.06211446335793));
#69461=CARTESIAN_POINT('',(-5.70356981034338,144.,9.15611397133807));
#69462=CARTESIAN_POINT('',(-5.70356981034338,144.,9.15611397133807));
#69463=CARTESIAN_POINT('',(-5.70356981034338,133.2,9.15611397133807));
#69464=CARTESIAN_POINT('',(-5.70356981034338,133.2,9.15611397133807));
#69465=CARTESIAN_POINT('',(-5.70356981034338,133.2,9.15611397133807));
#69466=CARTESIAN_POINT('Origin',(-6.00695118323399,133.2,8.93569450172839));
#69467=CARTESIAN_POINT('',(-5.9426404019167,133.2,8.72451914510537));
#69468=CARTESIAN_POINT('Origin',(0.,133.2,13.3));
#69469=CARTESIAN_POINT('',(-6.10460771782223,133.2,8.43211908408748));
#69470=CARTESIAN_POINT('Origin',(-5.70356981034338,133.2,9.15611397133807));
#69471=CARTESIAN_POINT('',(-5.9426404019167,144.,8.72451914510537));
#69472=CARTESIAN_POINT('',(-5.9426404019167,138.6,8.72451914510537));
#69473=CARTESIAN_POINT('',(-6.10460771782223,144.,8.43211908408748));
#69474=CARTESIAN_POINT('Origin',(-6.00695118323399,144.,8.93569450172839));
#69475=CARTESIAN_POINT('Origin',(0.,144.,13.3));
#69476=CARTESIAN_POINT('Origin',(-7.10874756357811,133.2,10.0707263854975));
#69477=CARTESIAN_POINT('',(-6.77468557884867,144.,10.0822934708492));
#69478=CARTESIAN_POINT('',(-6.77468557884867,133.2,10.0822934708492));
#69479=CARTESIAN_POINT('',(-6.77468557884867,138.6,10.0822934708492));
#69480=CARTESIAN_POINT('',(-6.28159599552799,144.,10.0993669768362));
#69481=CARTESIAN_POINT('',(-6.28159599552799,144.,10.0993669768362));
#69482=CARTESIAN_POINT('',(-6.28159599552799,133.2,10.0993669768362));
#69483=CARTESIAN_POINT('',(-6.28159599552799,133.2,10.0993669768362));
#69484=CARTESIAN_POINT('',(-6.28159599552799,133.2,10.0993669768362));
#69485=CARTESIAN_POINT('Origin',(-6.61572344209863,133.2,9.92912053943387));
#69486=CARTESIAN_POINT('',(-6.58523953715999,133.2,9.7104846792046));
#69487=CARTESIAN_POINT('Origin',(0.,133.2,13.3));
#69488=CARTESIAN_POINT('',(-6.79095421376043,133.2,9.44702181856561));
#69489=CARTESIAN_POINT('Origin',(-6.28159599552799,133.2,10.0993669768362));
#69490=CARTESIAN_POINT('',(-6.58523953715999,144.,9.7104846792046));
#69491=CARTESIAN_POINT('',(-6.58523953715999,138.6,9.7104846792046));
#69492=CARTESIAN_POINT('',(-6.79095421376043,144.,9.44702181856561));
#69493=CARTESIAN_POINT('Origin',(-6.61572344209863,144.,9.92912053943387));
#69494=CARTESIAN_POINT('Origin',(0.,144.,13.3));
#69495=CARTESIAN_POINT('Origin',(-7.52639677513343,133.2,11.2225372245787));
#69496=CARTESIAN_POINT('',(-7.19463815697102,144.,11.1817030920438));
#69497=CARTESIAN_POINT('',(-7.19463815697102,133.2,11.1817030920438));
#69498=CARTESIAN_POINT('',(-7.19463815697102,138.6,11.1817030920438));
#69499=CARTESIAN_POINT('',(-6.70494843988083,144.,11.1214301896566));
#69500=CARTESIAN_POINT('',(-6.70494843988083,144.,11.1214301896566));
#69501=CARTESIAN_POINT('',(-6.70494843988083,133.2,11.1214301896566));
#69502=CARTESIAN_POINT('',(-6.70494843988083,133.2,11.1214301896566));
#69503=CARTESIAN_POINT('',(-6.70494843988083,133.2,11.1214301896566));
#69504=CARTESIAN_POINT('Origin',(-7.06159463349151,133.2,11.005548816766));
#69505=CARTESIAN_POINT('',(-7.06568821984138,133.2,10.7848359934202));
#69506=CARTESIAN_POINT('Origin',(0.,133.2,13.3));
#69507=CARTESIAN_POINT('',(-7.31008487907097,133.2,10.5567976631721));
#69508=CARTESIAN_POINT('Origin',(-6.70494843988083,133.2,11.1214301896566));
#69509=CARTESIAN_POINT('',(-7.06568821984138,144.,10.7848359934202));
#69510=CARTESIAN_POINT('',(-7.06568821984138,138.6,10.7848359934202));
#69511=CARTESIAN_POINT('',(-7.31008487907097,144.,10.5567976631721));
#69512=CARTESIAN_POINT('Origin',(-7.06159463349151,144.,11.005548816766));
#69513=CARTESIAN_POINT('Origin',(0.,144.,13.3));
#69514=CARTESIAN_POINT('Origin',(-7.75872111940616,133.2,12.4255020918945));
#69515=CARTESIAN_POINT('',(-7.43743486603367,144.,12.3332722133368));
#69516=CARTESIAN_POINT('',(-7.43743486603367,133.2,12.3332722133368));
#69517=CARTESIAN_POINT('',(-7.43743486603367,138.6,12.3332722133368));
#69518=CARTESIAN_POINT('',(-6.96320280119572,144.,12.1971370214664));
#69519=CARTESIAN_POINT('',(-6.96320280119572,144.,12.1971370214664));
#69520=CARTESIAN_POINT('',(-6.96320280119572,133.2,12.1971370214664));
#69521=CARTESIAN_POINT('',(-6.96320280119572,133.2,12.1971370214664));
#69522=CARTESIAN_POINT('',(-6.96320280119572,133.2,12.1971370214664));
#69523=CARTESIAN_POINT('Origin',(-7.3335859289189,133.2,12.1384740970763));
#69524=CARTESIAN_POINT('',(-7.37215620887551,133.2,11.9211189928285));
#69525=CARTESIAN_POINT('Origin',(0.,133.2,13.3));
#69526=CARTESIAN_POINT('',(-7.64921699387799,133.2,11.7341202534779));
#69527=CARTESIAN_POINT('Origin',(-6.96320280119572,133.2,12.1971370214664));
#69528=CARTESIAN_POINT('',(-7.37215620887551,144.,11.9211189928285));
#69529=CARTESIAN_POINT('',(-7.37215620887551,138.6,11.9211189928285));
#69530=CARTESIAN_POINT('',(-7.64921699387799,144.,11.7341202534779));
#69531=CARTESIAN_POINT('Origin',(-7.3335859289189,144.,12.1384740970763));
#69532=CARTESIAN_POINT('Origin',(0.,144.,13.3));
#69533=CARTESIAN_POINT('Origin',(-7.8,133.2,13.65));
#69534=CARTESIAN_POINT('',(-7.4970972452634,144.,13.5086453811229));
#69535=CARTESIAN_POINT('',(-7.4970972452634,133.2,13.5086453811229));
#69536=CARTESIAN_POINT('',(-7.4970972452634,138.6,13.5086453811229));
#69537=CARTESIAN_POINT('',(-7.05,144.,13.3));
#69538=CARTESIAN_POINT('',(-7.05,144.,13.3));
#69539=CARTESIAN_POINT('',(-7.05,133.2,13.3));
#69540=CARTESIAN_POINT('',(-7.05,133.2,13.3));
#69541=CARTESIAN_POINT('',(-7.05,133.2,13.3));
#69542=CARTESIAN_POINT('Origin',(-7.425,133.2,13.3));
#69543=CARTESIAN_POINT('',(-7.5,133.2,13.3));
#69544=CARTESIAN_POINT('Origin',(0.,133.2,13.3));
#69545=CARTESIAN_POINT('',(-7.4970972452634,133.2,13.0913546188771));
#69546=CARTESIAN_POINT('',(-7.8,133.2,12.95));
#69547=CARTESIAN_POINT('Origin',(0.,133.2,13.3));
#69548=CARTESIAN_POINT('Origin',(-7.05,133.2,13.3));
#69549=CARTESIAN_POINT('',(-7.4970972452634,144.,13.0913546188771));
#69550=CARTESIAN_POINT('',(-7.4970972452634,138.6,13.0913546188771));
#69551=CARTESIAN_POINT('',(-7.8,144.,12.95));
#69552=CARTESIAN_POINT('Origin',(-7.425,144.,13.3));
#69553=CARTESIAN_POINT('',(-7.5,144.,13.3));
#69554=CARTESIAN_POINT('Origin',(0.,144.,13.3));
#69555=CARTESIAN_POINT('Origin',(0.,144.,13.3));
#69556=CARTESIAN_POINT('Origin',(-7.64921699387799,133.2,14.8658797465221));
#69557=CARTESIAN_POINT('',(-7.37215620887551,144.,14.6788810071715));
#69558=CARTESIAN_POINT('',(-7.37215620887551,133.2,14.6788810071715));
#69559=CARTESIAN_POINT('',(-7.37215620887551,138.6,14.6788810071715));
#69560=CARTESIAN_POINT('',(-6.96320280119572,144.,14.4028629785336));
#69561=CARTESIAN_POINT('',(-6.96320280119572,144.,14.4028629785336));
#69562=CARTESIAN_POINT('',(-6.96320280119572,133.2,14.4028629785336));
#69563=CARTESIAN_POINT('',(-6.96320280119572,133.2,14.4028629785336));
#69564=CARTESIAN_POINT('',(-6.96320280119572,133.2,14.4028629785336));
#69565=CARTESIAN_POINT('Origin',(-7.3335859289189,133.2,14.4615259029237));
#69566=CARTESIAN_POINT('',(-7.43743486603367,133.2,14.2667277866632));
#69567=CARTESIAN_POINT('Origin',(0.,133.2,13.3));
#69568=CARTESIAN_POINT('',(-7.75872111940616,133.2,14.1744979081055));
#69569=CARTESIAN_POINT('Origin',(-6.96320280119572,133.2,14.4028629785336));
#69570=CARTESIAN_POINT('',(-7.43743486603367,144.,14.2667277866632));
#69571=CARTESIAN_POINT('',(-7.43743486603367,138.6,14.2667277866632));
#69572=CARTESIAN_POINT('',(-7.75872111940616,144.,14.1744979081055));
#69573=CARTESIAN_POINT('Origin',(-7.3335859289189,144.,14.4615259029237));
#69574=CARTESIAN_POINT('Origin',(0.,144.,13.3));
#69575=CARTESIAN_POINT('Origin',(-7.31008487907097,133.2,16.0432023368279));
#69576=CARTESIAN_POINT('',(-7.06568821984138,144.,15.8151640065798));
#69577=CARTESIAN_POINT('',(-7.06568821984138,133.2,15.8151640065798));
#69578=CARTESIAN_POINT('',(-7.06568821984138,138.6,15.8151640065798));
#69579=CARTESIAN_POINT('',(-6.70494843988083,144.,15.4785698103434));
#69580=CARTESIAN_POINT('',(-6.70494843988083,144.,15.4785698103434));
#69581=CARTESIAN_POINT('',(-6.70494843988083,133.2,15.4785698103434));
#69582=CARTESIAN_POINT('',(-6.70494843988083,133.2,15.4785698103434));
#69583=CARTESIAN_POINT('',(-6.70494843988083,133.2,15.4785698103434));
#69584=CARTESIAN_POINT('Origin',(-7.06159463349151,133.2,15.594451183234));
#69585=CARTESIAN_POINT('',(-7.19463815697102,133.2,15.4182969079562));
#69586=CARTESIAN_POINT('Origin',(0.,133.2,13.3));
#69587=CARTESIAN_POINT('',(-7.52639677513343,133.2,15.3774627754213));
#69588=CARTESIAN_POINT('Origin',(-6.70494843988083,133.2,15.4785698103434));
#69589=CARTESIAN_POINT('',(-7.19463815697102,144.,15.4182969079562));
#69590=CARTESIAN_POINT('',(-7.19463815697102,138.6,15.4182969079562));
#69591=CARTESIAN_POINT('',(-7.52639677513343,144.,15.3774627754213));
#69592=CARTESIAN_POINT('Origin',(-7.06159463349151,144.,15.594451183234));
#69593=CARTESIAN_POINT('Origin',(0.,144.,13.3));
#69594=CARTESIAN_POINT('Origin',(-6.79095421376043,133.2,17.1529781814344));
#69595=CARTESIAN_POINT('',(-6.58523953715999,144.,16.8895153207954));
#69596=CARTESIAN_POINT('',(-6.58523953715999,133.2,16.8895153207954));
#69597=CARTESIAN_POINT('',(-6.58523953715999,138.6,16.8895153207954));
#69598=CARTESIAN_POINT('',(-6.28159599552799,144.,16.5006330231638));
#69599=CARTESIAN_POINT('',(-6.28159599552799,144.,16.5006330231638));
#69600=CARTESIAN_POINT('',(-6.28159599552799,133.2,16.5006330231638));
#69601=CARTESIAN_POINT('',(-6.28159599552799,133.2,16.5006330231638));
#69602=CARTESIAN_POINT('',(-6.28159599552799,133.2,16.5006330231638));
#69603=CARTESIAN_POINT('Origin',(-6.61572344209863,133.2,16.6708794605661));
#69604=CARTESIAN_POINT('',(-6.77468557884867,133.2,16.5177065291508));
#69605=CARTESIAN_POINT('Origin',(0.,133.2,13.3));
#69606=CARTESIAN_POINT('',(-7.10874756357811,133.2,16.5292736145025));
#69607=CARTESIAN_POINT('Origin',(-6.28159599552799,133.2,16.5006330231638));
#69608=CARTESIAN_POINT('',(-6.77468557884867,144.,16.5177065291508));
#69609=CARTESIAN_POINT('',(-6.77468557884867,138.6,16.5177065291508));
#69610=CARTESIAN_POINT('',(-7.10874756357811,144.,16.5292736145025));
#69611=CARTESIAN_POINT('Origin',(-6.61572344209863,144.,16.6708794605661));
#69612=CARTESIAN_POINT('Origin',(0.,144.,13.3));
#69613=CARTESIAN_POINT('Origin',(-6.10460771782222,133.2,18.1678809159125));
#69614=CARTESIAN_POINT('',(-5.9426404019167,144.,17.8754808548946));
#69615=CARTESIAN_POINT('',(-5.9426404019167,133.2,17.8754808548946));
#69616=CARTESIAN_POINT('',(-5.9426404019167,138.6,17.8754808548946));
#69617=CARTESIAN_POINT('',(-5.70356981034338,144.,17.4438860286619));
#69618=CARTESIAN_POINT('',(-5.70356981034338,144.,17.4438860286619));
#69619=CARTESIAN_POINT('',(-5.70356981034338,133.2,17.4438860286619));
#69620=CARTESIAN_POINT('',(-5.70356981034338,133.2,17.4438860286619));
#69621=CARTESIAN_POINT('',(-5.70356981034338,133.2,17.4438860286619));
#69622=CARTESIAN_POINT('Origin',(-6.00695118323398,133.2,17.6643054982716));
#69623=CARTESIAN_POINT('',(-6.18791775788269,133.2,17.5378855366421));
#69624=CARTESIAN_POINT('Origin',(0.,133.2,13.3));
#69625=CARTESIAN_POINT('',(-6.51605739442696,133.2,17.6015690198501));
#69626=CARTESIAN_POINT('Origin',(-5.70356981034338,133.2,17.4438860286619));
#69627=CARTESIAN_POINT('',(-6.18791775788269,144.,17.5378855366421));
#69628=CARTESIAN_POINT('',(-6.18791775788269,138.6,17.5378855366421));
#69629=CARTESIAN_POINT('',(-6.51605739442696,144.,17.6015690198501));
#69630=CARTESIAN_POINT('Origin',(-6.00695118323398,144.,17.6643054982716));
#69631=CARTESIAN_POINT('Origin',(0.,144.,13.3));
#69632=CARTESIAN_POINT('Origin',(-5.26794551983978,133.2,19.0629202666704));
#69633=CARTESIAN_POINT('',(-5.15371373748547,144.,18.748782865196));
#69634=CARTESIAN_POINT('',(-5.15371373748547,133.2,18.748782865196));
#69635=CARTESIAN_POINT('',(-5.15371373748547,138.6,18.748782865196));
#69636=CARTESIAN_POINT('',(-4.98510280736516,144.,18.2851028073652));
#69637=CARTESIAN_POINT('',(-4.98510280736516,144.,18.2851028073652));
#69638=CARTESIAN_POINT('',(-4.98510280736516,133.2,18.2851028073652));
#69639=CARTESIAN_POINT('',(-4.98510280736516,133.2,18.2851028073652));
#69640=CARTESIAN_POINT('',(-4.98510280736516,133.2,18.2851028073652));
#69641=CARTESIAN_POINT('Origin',(-5.25026785031011,133.2,18.5502678503101));
#69642=CARTESIAN_POINT('',(-5.44878286519601,133.2,18.4537137374855));
#69643=CARTESIAN_POINT('Origin',(0.,133.2,13.3));
#69644=CARTESIAN_POINT('',(-5.76292026667036,133.2,18.5679455198398));
#69645=CARTESIAN_POINT('Origin',(-4.98510280736516,133.2,18.2851028073652));
#69646=CARTESIAN_POINT('',(-5.44878286519601,144.,18.4537137374855));
#69647=CARTESIAN_POINT('',(-5.448782865196,138.6,18.4537137374855));
#69648=CARTESIAN_POINT('',(-5.76292026667036,144.,18.5679455198398));
#69649=CARTESIAN_POINT('Origin',(-5.25026785031011,144.,18.5502678503101));
#69650=CARTESIAN_POINT('Origin',(0.,144.,13.3));
#69651=CARTESIAN_POINT('Origin',(-4.30156901985006,133.2,19.816057394427));
#69652=CARTESIAN_POINT('',(-4.23788553664207,144.,19.4879177578827));
#69653=CARTESIAN_POINT('',(-4.23788553664207,133.2,19.4879177578827));
#69654=CARTESIAN_POINT('',(-4.23788553664207,138.6,19.4879177578827));
#69655=CARTESIAN_POINT('',(-4.14388602866194,144.,19.0035698103434));
#69656=CARTESIAN_POINT('',(-4.14388602866194,144.,19.0035698103434));
#69657=CARTESIAN_POINT('',(-4.14388602866194,133.2,19.0035698103434));
#69658=CARTESIAN_POINT('',(-4.14388602866194,133.2,19.0035698103434));
#69659=CARTESIAN_POINT('',(-4.14388602866194,133.2,19.0035698103434));
#69660=CARTESIAN_POINT('Origin',(-4.36430549827161,133.2,19.306951183234));
#69661=CARTESIAN_POINT('',(-4.57548085489463,133.2,19.2426404019167));
#69662=CARTESIAN_POINT('Origin',(0.,133.2,13.3));
#69663=CARTESIAN_POINT('',(-4.86788091591252,133.2,19.4046077178222));
#69664=CARTESIAN_POINT('Origin',(-4.14388602866194,133.2,19.0035698103434));
#69665=CARTESIAN_POINT('',(-4.57548085489463,144.,19.2426404019167));
#69666=CARTESIAN_POINT('',(-4.57548085489463,138.6,19.2426404019167));
#69667=CARTESIAN_POINT('',(-4.86788091591252,144.,19.4046077178222));
#69668=CARTESIAN_POINT('Origin',(-4.36430549827161,144.,19.306951183234));
#69669=CARTESIAN_POINT('Origin',(0.,144.,13.3));
#69670=CARTESIAN_POINT('Origin',(-3.22927361450253,133.2,20.4087475635781));
#69671=CARTESIAN_POINT('',(-3.21770652915082,144.,20.0746855788487));
#69672=CARTESIAN_POINT('',(-3.21770652915082,133.2,20.0746855788487));
#69673=CARTESIAN_POINT('',(-3.21770652915082,138.6,20.0746855788487));
#69674=CARTESIAN_POINT('',(-3.2006330231638,144.,19.581595995528));
#69675=CARTESIAN_POINT('',(-3.2006330231638,144.,19.581595995528));
#69676=CARTESIAN_POINT('',(-3.2006330231638,133.2,19.581595995528));
#69677=CARTESIAN_POINT('',(-3.2006330231638,133.2,19.581595995528));
#69678=CARTESIAN_POINT('',(-3.2006330231638,133.2,19.581595995528));
#69679=CARTESIAN_POINT('Origin',(-3.37087946056613,133.2,19.9157234420986));
#69680=CARTESIAN_POINT('',(-3.5895153207954,133.2,19.88523953716));
#69681=CARTESIAN_POINT('Origin',(0.,133.2,13.3));
#69682=CARTESIAN_POINT('',(-3.85297818143439,133.2,20.0909542137604));
#69683=CARTESIAN_POINT('Origin',(-3.2006330231638,133.2,19.581595995528));
#69684=CARTESIAN_POINT('',(-3.5895153207954,144.,19.88523953716));
#69685=CARTESIAN_POINT('',(-3.5895153207954,138.6,19.88523953716));
#69686=CARTESIAN_POINT('',(-3.85297818143439,144.,20.0909542137604));
#69687=CARTESIAN_POINT('Origin',(-3.37087946056613,144.,19.9157234420986));
#69688=CARTESIAN_POINT('Origin',(0.,144.,13.3));
#69689=CARTESIAN_POINT('Origin',(-2.07746277542129,133.2,20.8263967751334));
#69690=CARTESIAN_POINT('',(-2.11829690795615,144.,20.494638156971));
#69691=CARTESIAN_POINT('',(-2.11829690795615,133.2,20.494638156971));
#69692=CARTESIAN_POINT('',(-2.11829690795616,138.6,20.494638156971));
#69693=CARTESIAN_POINT('',(-2.17856981034338,144.,20.0049484398808));
#69694=CARTESIAN_POINT('',(-2.17856981034338,144.,20.0049484398808));
#69695=CARTESIAN_POINT('',(-2.17856981034338,133.2,20.0049484398808));
#69696=CARTESIAN_POINT('',(-2.17856981034338,133.2,20.0049484398808));
#69697=CARTESIAN_POINT('',(-2.17856981034338,133.2,20.0049484398808));
#69698=CARTESIAN_POINT('Origin',(-2.29445118323398,133.2,20.3615946334915));
#69699=CARTESIAN_POINT('',(-2.51516400657983,133.2,20.3656882198414));
#69700=CARTESIAN_POINT('Origin',(0.,133.2,13.3));
#69701=CARTESIAN_POINT('',(-2.74320233682789,133.2,20.610084879071));
#69702=CARTESIAN_POINT('Origin',(-2.17856981034338,133.2,20.0049484398808));
#69703=CARTESIAN_POINT('',(-2.51516400657983,144.,20.3656882198414));
#69704=CARTESIAN_POINT('',(-2.51516400657983,138.6,20.3656882198414));
#69705=CARTESIAN_POINT('',(-2.74320233682789,144.,20.610084879071));
#69706=CARTESIAN_POINT('Origin',(-2.29445118323398,144.,20.3615946334915));
#69707=CARTESIAN_POINT('Origin',(0.,144.,13.3));
#69708=CARTESIAN_POINT('Origin',(-0.874497908105503,133.2,21.0587211194062));
#69709=CARTESIAN_POINT('',(-0.966727786663231,144.,20.7374348660337));
#69710=CARTESIAN_POINT('',(-0.966727786663231,133.2,20.7374348660337));
#69711=CARTESIAN_POINT('',(-0.966727786663232,138.6,20.7374348660337));
#69712=CARTESIAN_POINT('',(-1.10286297853363,144.,20.2632028011957));
#69713=CARTESIAN_POINT('',(-1.10286297853363,144.,20.2632028011957));
#69714=CARTESIAN_POINT('',(-1.10286297853363,133.2,20.2632028011957));
#69715=CARTESIAN_POINT('',(-1.10286297853363,133.2,20.2632028011957));
#69716=CARTESIAN_POINT('',(-1.10286297853363,133.2,20.2632028011957));
#69717=CARTESIAN_POINT('Origin',(-1.16152590292371,133.2,20.6335859289189));
#69718=CARTESIAN_POINT('',(-1.37888100717151,133.2,20.6721562088755));
#69719=CARTESIAN_POINT('Origin',(0.,133.2,13.3));
#69720=CARTESIAN_POINT('',(-1.5658797465221,133.2,20.949216993878));
#69721=CARTESIAN_POINT('Origin',(-1.10286297853363,133.2,20.2632028011957));
#69722=CARTESIAN_POINT('',(-1.37888100717151,144.,20.6721562088755));
#69723=CARTESIAN_POINT('',(-1.37888100717151,138.6,20.6721562088755));
#69724=CARTESIAN_POINT('',(-1.5658797465221,144.,20.949216993878));
#69725=CARTESIAN_POINT('Origin',(-1.16152590292371,144.,20.6335859289189));
#69726=CARTESIAN_POINT('Origin',(0.,144.,13.3));
#69727=CARTESIAN_POINT('Origin',(0.349999999999999,133.2,21.1));
#69728=CARTESIAN_POINT('',(0.208645381122919,144.,20.7970972452634));
#69729=CARTESIAN_POINT('',(0.208645381122919,133.2,20.7970972452634));
#69730=CARTESIAN_POINT('',(0.208645381122919,138.6,20.7970972452634));
#69731=CARTESIAN_POINT('',(0.,144.,20.35));
#69732=CARTESIAN_POINT('',(0.,144.,20.35));
#69733=CARTESIAN_POINT('',(0.,133.2,20.35));
#69734=CARTESIAN_POINT('',(0.,133.2,20.35));
#69735=CARTESIAN_POINT('',(0.,133.2,20.35));
#69736=CARTESIAN_POINT('Origin',(0.,133.2,20.725));
#69737=CARTESIAN_POINT('',(-0.208645381122919,133.2,20.7970972452634));
#69738=CARTESIAN_POINT('Origin',(0.,133.2,13.3));
#69739=CARTESIAN_POINT('',(-0.349999999999999,133.2,21.1));
#69740=CARTESIAN_POINT('Origin',(0.,133.2,20.35));
#69741=CARTESIAN_POINT('',(-0.208645381122919,144.,20.7970972452634));
#69742=CARTESIAN_POINT('',(-0.208645381122919,138.6,20.7970972452634));
#69743=CARTESIAN_POINT('',(-0.349999999999999,144.,21.1));
#69744=CARTESIAN_POINT('Origin',(0.,144.,20.725));
#69745=CARTESIAN_POINT('Origin',(0.,144.,13.3));
#69746=CARTESIAN_POINT('Origin',(1.5658797465221,133.2,20.949216993878));
#69747=CARTESIAN_POINT('',(1.37888100717151,144.,20.6721562088755));
#69748=CARTESIAN_POINT('',(1.37888100717151,133.2,20.6721562088755));
#69749=CARTESIAN_POINT('',(1.37888100717151,138.6,20.6721562088755));
#69750=CARTESIAN_POINT('',(1.10286297853363,144.,20.2632028011957));
#69751=CARTESIAN_POINT('',(1.10286297853363,144.,20.2632028011957));
#69752=CARTESIAN_POINT('',(1.10286297853363,133.2,20.2632028011957));
#69753=CARTESIAN_POINT('',(1.10286297853363,133.2,20.2632028011957));
#69754=CARTESIAN_POINT('',(1.10286297853363,133.2,20.2632028011957));
#69755=CARTESIAN_POINT('Origin',(1.16152590292371,133.2,20.6335859289189));
#69756=CARTESIAN_POINT('',(0.966727786663231,133.2,20.7374348660337));
#69757=CARTESIAN_POINT('Origin',(0.,133.2,13.3));
#69758=CARTESIAN_POINT('',(0.874497908105503,133.2,21.0587211194062));
#69759=CARTESIAN_POINT('Origin',(1.10286297853363,133.2,20.2632028011957));
#69760=CARTESIAN_POINT('',(0.966727786663231,144.,20.7374348660337));
#69761=CARTESIAN_POINT('',(0.966727786663232,138.6,20.7374348660337));
#69762=CARTESIAN_POINT('',(0.874497908105503,144.,21.0587211194062));
#69763=CARTESIAN_POINT('Origin',(1.16152590292371,144.,20.6335859289189));
#69764=CARTESIAN_POINT('Origin',(0.,144.,13.3));
#69765=CARTESIAN_POINT('Origin',(2.74320233682789,133.2,20.610084879071));
#69766=CARTESIAN_POINT('',(2.51516400657983,144.,20.3656882198414));
#69767=CARTESIAN_POINT('',(2.51516400657983,133.2,20.3656882198414));
#69768=CARTESIAN_POINT('',(2.51516400657983,138.6,20.3656882198414));
#69769=CARTESIAN_POINT('',(2.17856981034338,144.,20.0049484398808));
#69770=CARTESIAN_POINT('',(2.17856981034338,144.,20.0049484398808));
#69771=CARTESIAN_POINT('',(2.17856981034338,133.2,20.0049484398808));
#69772=CARTESIAN_POINT('',(2.17856981034338,133.2,20.0049484398808));
#69773=CARTESIAN_POINT('',(2.17856981034338,133.2,20.0049484398808));
#69774=CARTESIAN_POINT('Origin',(2.29445118323399,133.2,20.3615946334915));
#69775=CARTESIAN_POINT('',(2.11829690795615,133.2,20.494638156971));
#69776=CARTESIAN_POINT('Origin',(0.,133.2,13.3));
#69777=CARTESIAN_POINT('',(2.07746277542129,133.2,20.8263967751334));
#69778=CARTESIAN_POINT('Origin',(2.17856981034338,133.2,20.0049484398808));
#69779=CARTESIAN_POINT('',(2.11829690795615,144.,20.494638156971));
#69780=CARTESIAN_POINT('',(2.11829690795616,138.6,20.494638156971));
#69781=CARTESIAN_POINT('',(2.07746277542129,144.,20.8263967751334));
#69782=CARTESIAN_POINT('Origin',(2.29445118323399,144.,20.3615946334915));
#69783=CARTESIAN_POINT('Origin',(0.,144.,13.3));
#69784=CARTESIAN_POINT('Origin',(3.85297818143439,133.2,20.0909542137604));
#69785=CARTESIAN_POINT('',(3.5895153207954,144.,19.88523953716));
#69786=CARTESIAN_POINT('',(3.5895153207954,133.2,19.88523953716));
#69787=CARTESIAN_POINT('',(3.5895153207954,138.6,19.88523953716));
#69788=CARTESIAN_POINT('',(3.20063302316381,144.,19.581595995528));
#69789=CARTESIAN_POINT('',(3.20063302316381,144.,19.581595995528));
#69790=CARTESIAN_POINT('',(3.20063302316381,133.2,19.581595995528));
#69791=CARTESIAN_POINT('',(3.20063302316381,133.2,19.581595995528));
#69792=CARTESIAN_POINT('',(3.20063302316381,133.2,19.581595995528));
#69793=CARTESIAN_POINT('Origin',(3.37087946056613,133.2,19.9157234420986));
#69794=CARTESIAN_POINT('',(3.21770652915082,133.2,20.0746855788487));
#69795=CARTESIAN_POINT('Origin',(0.,133.2,13.3));
#69796=CARTESIAN_POINT('',(3.22927361450254,133.2,20.4087475635781));
#69797=CARTESIAN_POINT('Origin',(3.20063302316381,133.2,19.581595995528));
#69798=CARTESIAN_POINT('',(3.21770652915082,144.,20.0746855788487));
#69799=CARTESIAN_POINT('',(3.21770652915082,138.6,20.0746855788487));
#69800=CARTESIAN_POINT('',(3.22927361450254,144.,20.4087475635781));
#69801=CARTESIAN_POINT('Origin',(3.37087946056613,144.,19.9157234420986));
#69802=CARTESIAN_POINT('Origin',(0.,144.,13.3));
#69803=CARTESIAN_POINT('Origin',(4.86788091591252,133.2,19.4046077178222));
#69804=CARTESIAN_POINT('',(4.57548085489463,144.,19.2426404019167));
#69805=CARTESIAN_POINT('',(4.57548085489463,133.2,19.2426404019167));
#69806=CARTESIAN_POINT('',(4.57548085489463,138.6,19.2426404019167));
#69807=CARTESIAN_POINT('',(4.14388602866194,144.,19.0035698103434));
#69808=CARTESIAN_POINT('',(4.14388602866194,144.,19.0035698103434));
#69809=CARTESIAN_POINT('',(4.14388602866194,133.2,19.0035698103434));
#69810=CARTESIAN_POINT('',(4.14388602866194,133.2,19.0035698103434));
#69811=CARTESIAN_POINT('',(4.14388602866194,133.2,19.0035698103434));
#69812=CARTESIAN_POINT('Origin',(4.36430549827161,133.2,19.306951183234));
#69813=CARTESIAN_POINT('',(4.23788553664207,133.2,19.4879177578827));
#69814=CARTESIAN_POINT('Origin',(0.,133.2,13.3));
#69815=CARTESIAN_POINT('',(4.30156901985006,133.2,19.816057394427));
#69816=CARTESIAN_POINT('Origin',(4.14388602866194,133.2,19.0035698103434));
#69817=CARTESIAN_POINT('',(4.23788553664207,144.,19.4879177578827));
#69818=CARTESIAN_POINT('',(4.23788553664207,138.6,19.4879177578827));
#69819=CARTESIAN_POINT('',(4.30156901985006,144.,19.816057394427));
#69820=CARTESIAN_POINT('Origin',(4.36430549827161,144.,19.306951183234));
#69821=CARTESIAN_POINT('Origin',(0.,144.,13.3));
#69822=CARTESIAN_POINT('Origin',(5.76292026667036,133.2,18.5679455198398));
#69823=CARTESIAN_POINT('',(5.44878286519601,144.,18.4537137374855));
#69824=CARTESIAN_POINT('',(5.44878286519601,133.2,18.4537137374855));
#69825=CARTESIAN_POINT('',(5.44878286519601,138.6,18.4537137374855));
#69826=CARTESIAN_POINT('',(4.98510280736516,144.,18.2851028073652));
#69827=CARTESIAN_POINT('',(4.98510280736516,144.,18.2851028073652));
#69828=CARTESIAN_POINT('',(4.98510280736516,133.2,18.2851028073652));
#69829=CARTESIAN_POINT('',(4.98510280736516,133.2,18.2851028073652));
#69830=CARTESIAN_POINT('',(4.98510280736516,133.2,18.2851028073652));
#69831=CARTESIAN_POINT('Origin',(5.25026785031011,133.2,18.5502678503101));
#69832=CARTESIAN_POINT('',(5.15371373748547,133.2,18.748782865196));
#69833=CARTESIAN_POINT('Origin',(0.,133.2,13.3));
#69834=CARTESIAN_POINT('',(5.26794551983978,133.2,19.0629202666704));
#69835=CARTESIAN_POINT('Origin',(4.98510280736516,133.2,18.2851028073652));
#69836=CARTESIAN_POINT('',(5.15371373748547,144.,18.748782865196));
#69837=CARTESIAN_POINT('',(5.15371373748547,138.6,18.748782865196));
#69838=CARTESIAN_POINT('',(5.26794551983978,144.,19.0629202666704));
#69839=CARTESIAN_POINT('Origin',(5.25026785031011,144.,18.5502678503101));
#69840=CARTESIAN_POINT('Origin',(0.,144.,13.3));
#69841=CARTESIAN_POINT('Origin',(6.51605739442696,133.2,17.6015690198501));
#69842=CARTESIAN_POINT('',(6.18791775788269,144.,17.5378855366421));
#69843=CARTESIAN_POINT('',(6.18791775788269,133.2,17.5378855366421));
#69844=CARTESIAN_POINT('',(6.18791775788269,138.6,17.5378855366421));
#69845=CARTESIAN_POINT('',(5.70356981034338,144.,17.4438860286619));
#69846=CARTESIAN_POINT('',(5.70356981034338,144.,17.4438860286619));
#69847=CARTESIAN_POINT('',(5.70356981034338,133.2,17.4438860286619));
#69848=CARTESIAN_POINT('',(5.70356981034338,133.2,17.4438860286619));
#69849=CARTESIAN_POINT('',(5.70356981034338,133.2,17.4438860286619));
#69850=CARTESIAN_POINT('Origin',(6.00695118323398,133.2,17.6643054982716));
#69851=CARTESIAN_POINT('',(5.9426404019167,133.2,17.8754808548946));
#69852=CARTESIAN_POINT('Origin',(0.,133.2,13.3));
#69853=CARTESIAN_POINT('',(6.10460771782223,133.2,18.1678809159125));
#69854=CARTESIAN_POINT('Origin',(5.70356981034338,133.2,17.4438860286619));
#69855=CARTESIAN_POINT('',(5.9426404019167,144.,17.8754808548946));
#69856=CARTESIAN_POINT('',(5.9426404019167,138.6,17.8754808548946));
#69857=CARTESIAN_POINT('',(6.10460771782223,144.,18.1678809159125));
#69858=CARTESIAN_POINT('Origin',(6.00695118323398,144.,17.6643054982716));
#69859=CARTESIAN_POINT('Origin',(0.,144.,13.3));
#69860=CARTESIAN_POINT('Origin',(7.10874756357811,133.2,16.5292736145025));
#69861=CARTESIAN_POINT('',(6.77468557884867,144.,16.5177065291508));
#69862=CARTESIAN_POINT('',(6.77468557884867,133.2,16.5177065291508));
#69863=CARTESIAN_POINT('',(6.77468557884867,138.6,16.5177065291508));
#69864=CARTESIAN_POINT('',(6.28159599552799,144.,16.5006330231638));
#69865=CARTESIAN_POINT('',(6.28159599552799,144.,16.5006330231638));
#69866=CARTESIAN_POINT('',(6.28159599552799,133.2,16.5006330231638));
#69867=CARTESIAN_POINT('',(6.28159599552799,133.2,16.5006330231638));
#69868=CARTESIAN_POINT('',(6.28159599552799,133.2,16.5006330231638));
#69869=CARTESIAN_POINT('Origin',(6.61572344209863,133.2,16.6708794605661));
#69870=CARTESIAN_POINT('',(6.58523953715999,133.2,16.8895153207954));
#69871=CARTESIAN_POINT('Origin',(0.,133.2,13.3));
#69872=CARTESIAN_POINT('',(6.79095421376043,133.2,17.1529781814344));
#69873=CARTESIAN_POINT('Origin',(6.28159599552799,133.2,16.5006330231638));
#69874=CARTESIAN_POINT('',(6.58523953715999,144.,16.8895153207954));
#69875=CARTESIAN_POINT('',(6.58523953715999,138.6,16.8895153207954));
#69876=CARTESIAN_POINT('',(6.79095421376043,144.,17.1529781814344));
#69877=CARTESIAN_POINT('Origin',(6.61572344209863,144.,16.6708794605661));
#69878=CARTESIAN_POINT('Origin',(0.,144.,13.3));
#69879=CARTESIAN_POINT('Origin',(7.52639677513343,133.2,15.3774627754213));
#69880=CARTESIAN_POINT('',(7.19463815697102,144.,15.4182969079562));
#69881=CARTESIAN_POINT('',(7.19463815697102,133.2,15.4182969079562));
#69882=CARTESIAN_POINT('',(7.19463815697102,138.6,15.4182969079562));
#69883=CARTESIAN_POINT('',(6.70494843988083,144.,15.4785698103434));
#69884=CARTESIAN_POINT('',(6.70494843988083,144.,15.4785698103434));
#69885=CARTESIAN_POINT('',(6.70494843988083,133.2,15.4785698103434));
#69886=CARTESIAN_POINT('',(6.70494843988083,133.2,15.4785698103434));
#69887=CARTESIAN_POINT('',(6.70494843988083,133.2,15.4785698103434));
#69888=CARTESIAN_POINT('Origin',(7.06159463349151,133.2,15.594451183234));
#69889=CARTESIAN_POINT('',(7.06568821984138,133.2,15.8151640065798));
#69890=CARTESIAN_POINT('Origin',(0.,133.2,13.3));
#69891=CARTESIAN_POINT('',(7.31008487907097,133.2,16.0432023368279));
#69892=CARTESIAN_POINT('Origin',(6.70494843988083,133.2,15.4785698103434));
#69893=CARTESIAN_POINT('',(7.06568821984138,144.,15.8151640065798));
#69894=CARTESIAN_POINT('',(7.06568821984138,138.6,15.8151640065798));
#69895=CARTESIAN_POINT('',(7.31008487907097,144.,16.0432023368279));
#69896=CARTESIAN_POINT('Origin',(7.06159463349151,144.,15.594451183234));
#69897=CARTESIAN_POINT('Origin',(0.,144.,13.3));
#69898=CARTESIAN_POINT('Origin',(7.75872111940616,133.2,14.1744979081055));
#69899=CARTESIAN_POINT('',(7.43743486603367,144.,14.2667277866632));
#69900=CARTESIAN_POINT('',(7.43743486603367,138.6,14.2667277866632));
#69901=CARTESIAN_POINT('',(6.96320280119572,144.,14.4028629785336));
#69902=CARTESIAN_POINT('',(6.96320280119572,144.,14.4028629785336));
#69903=CARTESIAN_POINT('',(6.96320280119572,133.2,14.4028629785336));
#69904=CARTESIAN_POINT('Origin',(7.3335859289189,133.2,14.4615259029237));
#69905=CARTESIAN_POINT('Origin',(0.,133.2,13.3));
#69906=CARTESIAN_POINT('Origin',(6.96320280119572,133.2,14.4028629785336));
#69907=CARTESIAN_POINT('',(7.37215620887551,144.,14.6788810071715));
#69908=CARTESIAN_POINT('',(7.64921699387799,144.,14.8658797465221));
#69909=CARTESIAN_POINT('',(7.37215620887551,138.6,14.6788810071715));
#69910=CARTESIAN_POINT('Origin',(7.3335859289189,144.,14.4615259029237));
#69911=CARTESIAN_POINT('Origin',(0.,144.,13.3));
#69912=CARTESIAN_POINT('Origin',(7.425,133.2,13.3));
#69913=CARTESIAN_POINT('Origin',(0.,133.2,13.3));
#69914=CARTESIAN_POINT('Origin',(7.425,144.,13.3));
#69915=CARTESIAN_POINT('Origin',(0.,144.,13.3));
#69916=CARTESIAN_POINT('Origin',(0.,144.95,13.3));
#69917=CARTESIAN_POINT('',(-2.01,144.7,13.3));
#69918=CARTESIAN_POINT('Origin',(0.,144.7,13.3));
#69919=CARTESIAN_POINT('',(-5.8,145.2,13.3));
#69920=CARTESIAN_POINT('',(-3.905,144.95,13.3));
#69921=CARTESIAN_POINT('Origin',(0.,145.2,13.3));
#69922=CARTESIAN_POINT('Origin',(6.9,145.2,13.3));
#69923=CARTESIAN_POINT('',(-6.9,145.2,13.3));
#69924=CARTESIAN_POINT('Origin',(0.,145.2,13.3));
#69925=CARTESIAN_POINT('Origin',(0.,144.9,13.3));
#69926=CARTESIAN_POINT('',(-7.5,144.6,13.3));
#69927=CARTESIAN_POINT('Origin',(0.,144.6,13.3));
#69928=CARTESIAN_POINT('',(-7.2,144.9,13.3));
#69929=CARTESIAN_POINT('Origin',(0.,138.6,13.3));
#69930=CARTESIAN_POINT('',(-7.5,132.6,13.3));
#69931=CARTESIAN_POINT('Origin',(0.,132.6,13.3));
#69932=CARTESIAN_POINT('',(-7.5,138.6,13.3));
#69933=CARTESIAN_POINT('',(-7.5,138.6,13.3));
#69934=CARTESIAN_POINT('Origin',(0.,132.4,13.3));
#69935=CARTESIAN_POINT('',(-7.1,132.2,13.3));
#69936=CARTESIAN_POINT('',(-7.3,132.4,13.3));
#69937=CARTESIAN_POINT('Origin',(0.,132.2,13.3));
#69938=CARTESIAN_POINT('Origin',(2.8,132.2,13.3));
#69939=CARTESIAN_POINT('',(-2.8,132.2,13.3));
#69940=CARTESIAN_POINT('Origin',(0.,132.2,13.3));
#69941=CARTESIAN_POINT('Origin',(0.,131.125,13.3));
#69942=CARTESIAN_POINT('',(-2.8,130.05,13.3));
#69943=CARTESIAN_POINT('Origin',(0.,130.05,13.3));
#69944=CARTESIAN_POINT('',(-2.8,131.125,13.3));
#69945=CARTESIAN_POINT('Origin',(2.01,130.05,13.3));
#69946=CARTESIAN_POINT('',(-2.01,130.05,13.3));
#69947=CARTESIAN_POINT('Origin',(0.,130.05,13.3));
#69948=CARTESIAN_POINT('Origin',(0.,137.625,13.3));
#69949=CARTESIAN_POINT('',(-2.01,137.625,13.3));
#135258=UNCERTAINTY_MEASURE_WITH_UNIT(LENGTH_MEASURE(0.01),#135283,
'DISTANCE_ACCURACY_VALUE',
'Maximum model space distance between geometric entities at asserted c
onnectivities');
#135267=UNCERTAINTY_MEASURE_WITH_UNIT(LENGTH_MEASURE(0.01),#135283,
'DISTANCE_ACCURACY_VALUE',
'Maximum model space distance between geometric entities at asserted c
onnectivities');
#135273=(
GEOMETRIC_REPRESENTATION_CONTEXT(3)
GLOBAL_UNCERTAINTY_ASSIGNED_CONTEXT((#135258))
GLOBAL_UNIT_ASSIGNED_CONTEXT((#135283,#135285,#135286))
REPRESENTATION_CONTEXT('','3D')
);
#135282=(
GEOMETRIC_REPRESENTATION_CONTEXT(3)
GLOBAL_UNCERTAINTY_ASSIGNED_CONTEXT((#135267))
GLOBAL_UNIT_ASSIGNED_CONTEXT((#135283,#135285,#135286))
REPRESENTATION_CONTEXT('','3D')
);
#135283=(
LENGTH_UNIT()
NAMED_UNIT(*)
SI_UNIT(.MILLI.,.METRE.)
);
#135285=(
NAMED_UNIT(*)
PLANE_ANGLE_UNIT()
SI_UNIT($,.RADIAN.)
);
#135286=(
NAMED_UNIT(*)
SI_UNIT($,.STERADIAN.)
SOLID_ANGLE_UNIT()
);
#135292=SHAPE_DEFINITION_REPRESENTATION(#135306,#135341);
#135306=PRODUCT_DEFINITION_SHAPE('',$,#135356);
#135341=SHAPE_REPRESENTATION('',(#32477),#135273);
#135350=PRODUCT_DEFINITION_CONTEXT('part definition',#135394,'design');
#135356=PRODUCT_DEFINITION('2026-10-15-19-09-11-260',
'Feed Knob D15 Knurled',#135370,#135350);
#135370=PRODUCT_DEFINITION_FORMATION('',$,#135401);
#135394=APPLICATION_CONTEXT(
'Core Data for Automotive Mechanical Design Process');
#135395=PRODUCT_CONTEXT('part definition',#135394,'mechanical');
#135401=PRODUCT('2026-10-15-19-09-11-260','Feed Knob D15 Knurled',$,(#135395));
#135415=PRESENTATION_STYLE_ASSIGNMENT((#135429));
#135429=SURFACE_STYLE_USAGE(.BOTH.,#135443);
#135443=SURFACE_SIDE_STYLE('',(#135457));
#135457=SURFACE_STYLE_FILL_AREA(#135471);
#135471=FILL_AREA_STYLE('Opaque(228,231,235)',(#135485));
#135485=FILL_AREA_STYLE_COLOUR('Opaque(228,231,235)',#135499);
#135499=COLOUR_RGB('Opaque(228,231,235)', 0.72549020, 0.75294118, 0.79215686);
ENDSEC;
END-ISO-10303-21;
